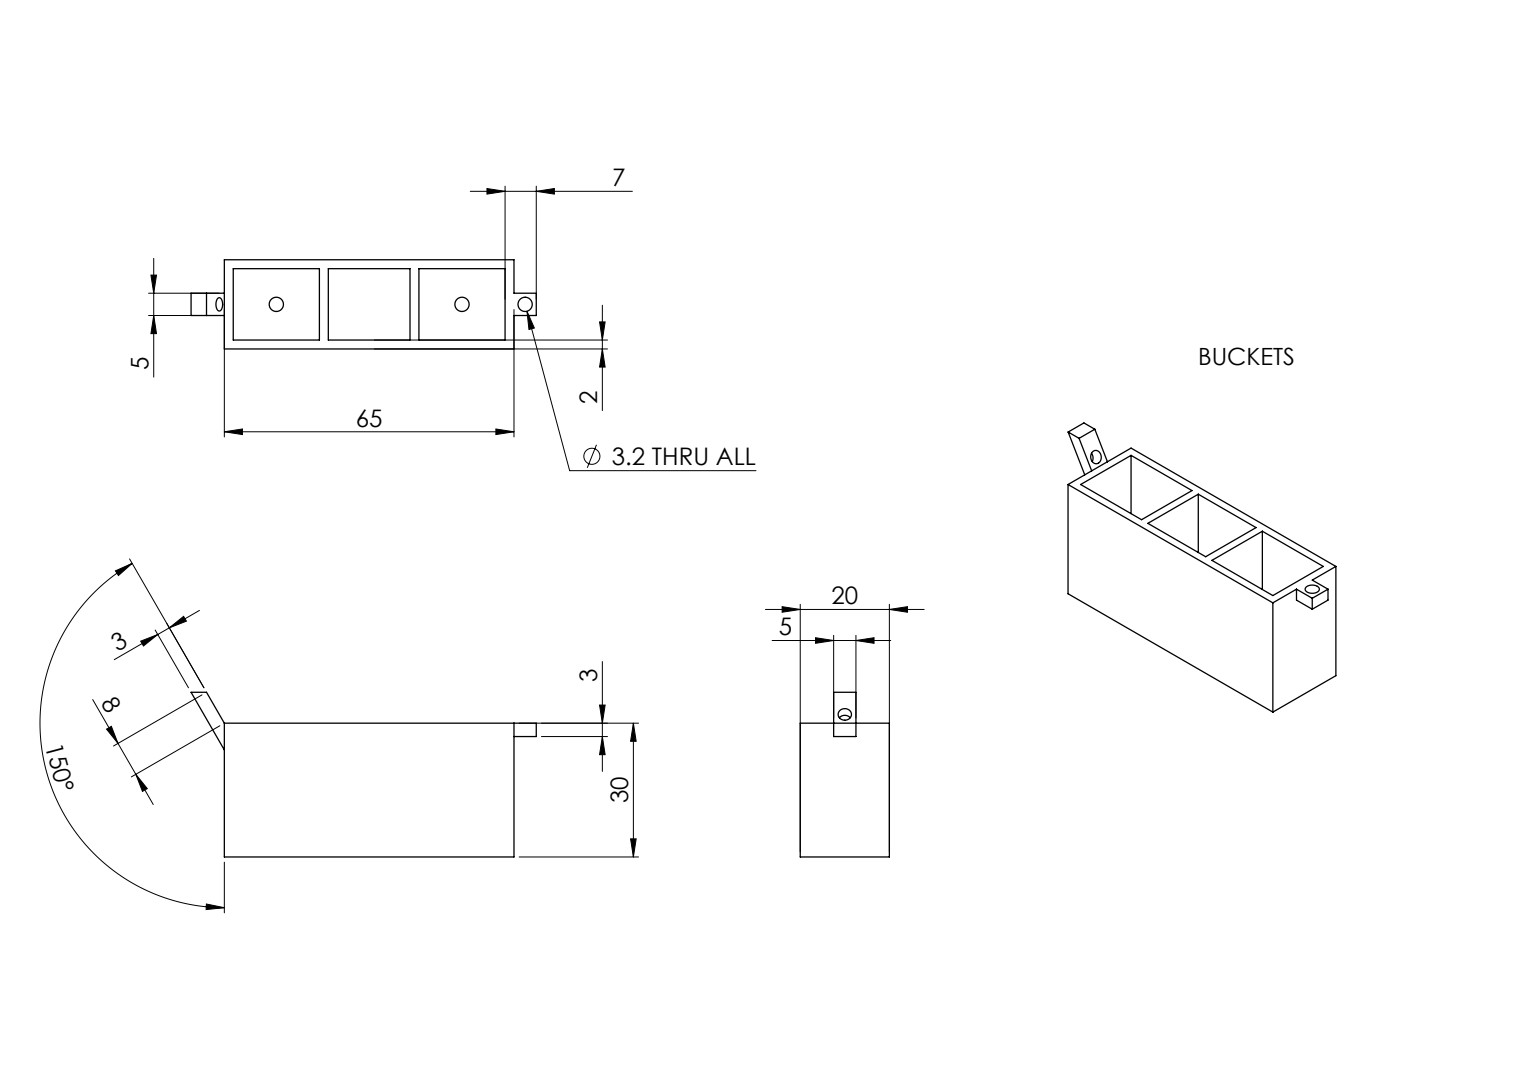
ISO-10303-21;
HEADER;
FILE_DESCRIPTION (('STEP AP214'),
    '1' );
FILE_NAME ('buckets.step',
    '2026-10-26T05:17:54',
    ( '' ),
    ( '' ),
    'SwSTEP 2.0',
    'SolidWorks 2026',
    '' );
FILE_SCHEMA (( 'AUTOMOTIVE_DESIGN' ));
ENDSEC;

DATA;
#10=VECTOR ( 'NONE', #6065, 1000.000000000000000 ) ;
#11=CARTESIAN_POINT ( 'NONE',  ( -6.666666666666660745, 2.000000000000001332, 1.599999999999986766 ) ) ;
#16=EDGE_CURVE ( 'NONE', #1898, #4275, #11568, .T. ) ;
#53=FACE_OUTER_BOUND ( 'NONE', #7053, .T. ) ;
#59=EDGE_CURVE ( 'NONE', #10107, #9996, #12197, .T. ) ;
#63=DIRECTION ( 'NONE',  ( 0.000000000000000000, 0.000000000000000000, 1.000000000000000000 ) ) ;
#76=AXIS2_PLACEMENT_3D ( 'NONE', #9120, #143, #2199 ) ;
#79=CARTESIAN_POINT ( 'NONE',  ( 9.999999999999994671, 27.00000000000000000, -2.500000000000000000 ) ) ;
#89=CARTESIAN_POINT ( 'NONE',  ( -63.73205080756886076, 30.46410161513775350, 0.000000000000000000 ) ) ;
#93=DIRECTION ( 'NONE',  ( -1.000000000000000000, 0.000000000000000000, -5.337610695313252124E-17 ) ) ;
#101=CYLINDRICAL_SURFACE ( 'NONE', #2852, 1.500000000000002665 ) ;
#104=ORIENTED_EDGE ( 'NONE', *, *, #6904, .F. ) ;
#116=ORIENTED_EDGE ( 'NONE', *, *, #12848, .F. ) ;
#143=DIRECTION ( 'NONE',  ( 0.8660254037844394848, 0.4999999999999985012, -0.000000000000000000 ) ) ;
#148=VECTOR ( 'NONE', #2125, 1000.000000000000000 ) ;
#152=( NAMED_UNIT ( * ) SI_UNIT ( $, .STERADIAN. ) SOLID_ANGLE_UNIT ( ) );
#153=DIRECTION ( 'NONE',  ( 1.000000000000000000, 0.000000000000000000, 0.000000000000000000 ) ) ;
#154=CARTESIAN_POINT ( 'NONE',  ( -16.33333333333332504, 2.000000000000000000, -7.999999999999996447 ) ) ;
#177=AXIS2_PLACEMENT_3D ( 'NONE', #10077, #4014, #1048 ) ;
#192=LINE ( 'NONE', #5111, #8966 ) ;
#205=AXIS2_PLACEMENT_3D ( 'NONE', #12610, #4630, #6775 ) ;
#217=FILL_AREA_STYLE ('',( #283 ) ) ;
#220=LINE ( 'NONE', #6117, #2380 ) ;
#231=VECTOR ( 'NONE', #9140, 1000.000000000000000 ) ;
#256=DIRECTION ( 'NONE',  ( 0.000000000000000000, 0.000000000000000000, 1.000000000000000000 ) ) ;
#273=CARTESIAN_POINT ( 'NONE',  ( -60.00000000000000000, 23.99999999999998934, 2.500000000000000000 ) ) ;
#283=FILL_AREA_STYLE_COLOUR ( '', #7592 ) ;
#286=FACE_OUTER_BOUND ( 'NONE', #5183, .T. ) ;
#289=EDGE_LOOP ( 'NONE', ( #1284, #1485, #7281, #1532 ) ) ;
#319=LINE ( 'NONE', #8516, #3101 ) ;
#347=DIRECTION ( 'NONE',  ( -0.000000000000000000, 1.000000000000000000, -0.000000000000000000 ) ) ;
#351=ADVANCED_FACE ( 'NONE', ( #11353 ), #2405, .T. ) ;
#357=DIRECTION ( 'NONE',  ( -1.000000000000000000, -0.000000000000000000, -0.000000000000000000 ) ) ;
#378=ORIENTED_EDGE ( 'NONE', *, *, #6492, .T. ) ;
#381=FACE_BOUND ( 'NONE', #9201, .T. ) ;
#386=DIRECTION ( 'NONE',  ( -0.000000000000000000, 1.000000000000000000, -0.000000000000000000 ) ) ;
#406=LINE ( 'NONE', #4420, #3286 ) ;
#419=EDGE_CURVE ( 'NONE', #6987, #1436, #9061, .T. ) ;
#436=ORIENTED_EDGE ( 'NONE', *, *, #12848, .T. ) ;
#445=ORIENTED_EDGE ( 'NONE', *, *, #1486, .T. ) ;
#446=CARTESIAN_POINT ( 'NONE',  ( 0.000000000000000000, 2.000000000000000000, 0.000000000000000000 ) ) ;
#448=VECTOR ( 'NONE', #5301, 1000.000000000000000 ) ;
#449=ORIENTED_EDGE ( 'NONE', *, *, #16, .T. ) ;
#452=DIRECTION ( 'NONE',  ( -0.000000000000000000, -1.000000000000000000, -0.000000000000000000 ) ) ;
#498=ORIENTED_EDGE ( 'NONE', *, *, #4803, .F. ) ;
#513=ORIENTED_EDGE ( 'NONE', *, *, #12102, .F. ) ;
#524=ORIENTED_EDGE ( 'NONE', *, *, #12861, .T. ) ;
#533=VECTOR ( 'NONE', #6646, 1000.000000000000000 ) ;
#534=DIRECTION ( 'NONE',  ( 0.4999999999999987232, -0.8660254037844393737, 0.000000000000000000 ) ) ;
#544=LINE ( 'NONE', #8546, #10 ) ;
#551=DIRECTION ( 'NONE',  ( -0.000000000000000000, -1.000000000000000000, -0.000000000000000000 ) ) ;
#569=AXIS2_PLACEMENT_3D ( 'NONE', #2591, #4682, #2724 ) ;
#573=SHAPE_DEFINITION_REPRESENTATION ( #2509, #985 ) ;
#585=VERTEX_POINT ( 'NONE', #1932 ) ;
#590=ORIENTED_EDGE ( 'NONE', *, *, #5677, .T. ) ;
#597=DIRECTION ( 'NONE',  ( -0.000000000000000000, -1.000000000000000000, -0.000000000000000000 ) ) ;
#604=CARTESIAN_POINT ( 'NONE',  ( -6.666666666666660745, 2.000000000000001332, -1.599999999999986766 ) ) ;
#605=VECTOR ( 'NONE', #12118, 1000.000000000000000 ) ;
#608=VECTOR ( 'NONE', #6526, 1000.000000000000000 ) ;
#616=VECTOR ( 'NONE', #1823, 1000.000000000000000 ) ;
#635=DIRECTION ( 'NONE',  ( -1.000000000000000000, 0.000000000000000000, 0.000000000000000000 ) ) ;
#637=DIRECTION ( 'NONE',  ( 0.000000000000000000, 0.000000000000000000, -1.000000000000000000 ) ) ;
#649=LINE ( 'NONE', #2821, #9778 ) ;
#654=CARTESIAN_POINT ( 'NONE',  ( -60.00000000000000000, 30.00000000000000000, 2.500000000000000000 ) ) ;
#669=VECTOR ( 'NONE', #1046, 1000.000000000000000 ) ;
#677=VECTOR ( 'NONE', #9665, 1000.000000000000000 ) ;
#688=CARTESIAN_POINT ( 'NONE',  ( 7.500000000000000000, 27.00000000000000000, 0.000000000000000000 ) ) ;
#697=CARTESIAN_POINT ( 'NONE',  ( 0.000000000000000000, 2.000000000000000000, 0.000000000000000000 ) ) ;
#703=VERTEX_POINT ( 'NONE', #4159 ) ;
#712=LINE ( 'NONE', #12759, #4156 ) ;
#720=EDGE_LOOP ( 'NONE', ( #4308, #11552, #5164, #9758 ) ) ;
#727=CARTESIAN_POINT ( 'NONE',  ( -60.00000000000000000, 30.00000000000000000, 9.999999999999996447 ) ) ;
#734=CIRCLE ( 'NONE', #6785, 1.599999999999997202 ) ;
#747=EDGE_CURVE ( 'NONE', #10649, #11707, #5061, .T. ) ;
#751=CARTESIAN_POINT ( 'NONE',  ( 5.000000000000004441, 30.00000000000000000, -2.500000000000000444 ) ) ;
#762=DIRECTION ( 'NONE',  ( -0.000000000000000000, -1.000000000000000000, -0.000000000000000000 ) ) ;
#764=DIRECTION ( 'NONE',  ( -1.000000000000000000, 0.000000000000000000, 0.000000000000000000 ) ) ;
#774=ADVANCED_FACE ( 'NONE', ( #8212, #1329 ), #3249, .F. ) ;
#782=ORIENTED_EDGE ( 'NONE', *, *, #419, .T. ) ;
#788=DIRECTION ( 'NONE',  ( -0.000000000000000000, 1.000000000000000000, -0.000000000000000000 ) ) ;
#792=CIRCLE ( 'NONE', #10416, 1.599999999999992095 ) ;
#793=CARTESIAN_POINT ( 'NONE',  ( -57.99999999999999289, 30.00000000000000000, -8.000000000000003553 ) ) ;
#794=EDGE_CURVE ( 'NONE', #11167, #1351, #9250, .T. ) ;
#826=DIRECTION ( 'NONE',  ( 0.5000000000000005551, -0.8660254037844383745, 0.000000000000000000 ) ) ;
#846=EDGE_LOOP ( 'NONE', ( #6406, #7183, #10691, #3671 ) ) ;
#848=CARTESIAN_POINT ( 'NONE',  ( 0.000000000000000000, 2.000000000000000000, 0.000000000000000000 ) ) ;
#861=EDGE_LOOP ( 'NONE', ( #5404, #2432, #3556, #8105 ) ) ;
#876=CARTESIAN_POINT ( 'NONE',  ( -38.66666666666665719, 30.00000000000000000, -7.999999999999996447 ) ) ;
#884=LINE ( 'NONE', #4888, #12292 ) ;
#895=EDGE_CURVE ( 'NONE', #11453, #7103, #8540, .T. ) ;
#899=PLANE ( 'NONE',  #11027 ) ;
#907=ORIENTED_EDGE ( 'NONE', *, *, #8637, .T. ) ;
#915=FACE_OUTER_BOUND ( 'NONE', #12172, .T. ) ;
#919=VERTEX_POINT ( 'NONE', #604 ) ;
#923=LINE ( 'NONE', #4988, #10114 ) ;
#941=AXIS2_PLACEMENT_3D ( 'NONE', #12279, #5334, #12079 ) ;
#944=ORIENTED_EDGE ( 'NONE', *, *, #9425, .F. ) ;
#946=VERTEX_POINT ( 'NONE', #11338 ) ;
#959=ORIENTED_EDGE ( 'NONE', *, *, #12861, .F. ) ;
#985=SHAPE_REPRESENTATION ( 'buckets', ( #5704 ), #1096 ) ;
#994=EDGE_CURVE ( 'NONE', #5904, #1184, #923, .T. ) ;
#1000=CARTESIAN_POINT ( 'NONE',  ( 4.270088556250601699E-16, 30.00000000000000000, -8.000000000000000000 ) ) ;
#1007=DIRECTION ( 'NONE',  ( -0.000000000000000000, 0.000000000000000000, 1.000000000000000000 ) ) ;
#1028=ORIENTED_EDGE ( 'NONE', *, *, #8827, .F. ) ;
#1032=CARTESIAN_POINT ( 'NONE',  ( 3.000000000000004441, 30.00000000000000000, -10.00000000000000000 ) ) ;
#1037=ORIENTED_EDGE ( 'NONE', *, *, #2209, .F. ) ;
#1046=DIRECTION ( 'NONE',  ( -0.000000000000000000, 1.000000000000000000, -0.000000000000000000 ) ) ;
#1048=DIRECTION ( 'NONE',  ( -1.000000000000000000, 0.000000000000000000, -5.337610695313252124E-17 ) ) ;
#1057=ORIENTED_EDGE ( 'NONE', *, *, #4752, .T. ) ;
#1070=STYLED_ITEM('',(#12995),#11791);
#1078=SURFACE_STYLE_FILL_AREA ( #217 ) ;
#1083=ORIENTED_EDGE ( 'NONE', *, *, #11509, .F. ) ;
#1085=DIRECTION ( 'NONE',  ( -0.000000000000000000, -1.000000000000000000, -0.000000000000000000 ) ) ;
#1088=CARTESIAN_POINT ( 'NONE',  ( -63.99999999999998579, 36.92820323027551410, -2.500000000000000000 ) ) ;
#1094=PLANE ( 'NONE',  #2692 ) ;
#1096=( GEOMETRIC_REPRESENTATION_CONTEXT ( 3 ) GLOBAL_UNCERTAINTY_ASSIGNED_CONTEXT ( ( #6479 ) ) GLOBAL_UNIT_ASSIGNED_CONTEXT ( ( #3190, #9328, #152 ) ) REPRESENTATION_CONTEXT ( 'NONE', 'WORKASPACE' ) );
#1117=DIRECTION ( 'NONE',  ( 0.000000000000000000, 1.000000000000000000, 0.000000000000000000 ) ) ;
#1143=EDGE_LOOP ( 'NONE', ( #5966, #12184, #3162, #12895 ) ) ;
#1153=EDGE_CURVE ( 'NONE', #2281, #8808, #11372, .T. ) ;
#1164=DIRECTION ( 'NONE',  ( 0.000000000000000000, 0.000000000000000000, -1.000000000000000000 ) ) ;
#1184=VERTEX_POINT ( 'NONE', #10716 ) ;
#1221=CARTESIAN_POINT ( 'NONE',  ( -60.38397459621555186, 30.66506350946108128, 0.000000000000000000 ) ) ;
#1228=PLANE ( 'NONE',  #11328 ) ;
#1243=DIRECTION ( 'NONE',  ( -0.000000000000000000, -1.000000000000000000, -0.000000000000000000 ) ) ;
#1247=FACE_BOUND ( 'NONE', #3736, .T. ) ;
#1251=CARTESIAN_POINT ( 'NONE',  ( -48.33333333333332860, 2.000000000000001332, -1.599999999999992095 ) ) ;
#1284=ORIENTED_EDGE ( 'NONE', *, *, #4752, .F. ) ;
#1286=CARTESIAN_POINT ( 'NONE',  ( -61.88397459621555186, 33.26313972081440085, 1.836970198721030427E-16 ) ) ;
#1294=CARTESIAN_POINT ( 'NONE',  ( -60.00000000000000000, 30.00000000000000000, 7.999999999999996447 ) ) ;
#1298=VECTOR ( 'NONE', #9824, 1000.000000000000000 ) ;
#1300=EDGE_LOOP ( 'NONE', ( #9011, #8775, #11719, #6124 ) ) ;
#1305=ORIENTED_EDGE ( 'NONE', *, *, #12229, .T. ) ;
#1309=CARTESIAN_POINT ( 'NONE',  ( 9.999999999999994671, 30.00000000000000000, -2.500000000000000000 ) ) ;
#1312=ORIENTED_EDGE ( 'NONE', *, *, #1891, .T. ) ;
#1319=CARTESIAN_POINT ( 'NONE',  ( -67.46410161513773573, 36.92820323027551410, 2.500000000000000000 ) ) ;
#1329=FACE_OUTER_BOUND ( 'NONE', #9005, .T. ) ;
#1330=DIRECTION ( 'NONE',  ( 1.000000000000000000, 0.000000000000000000, 5.337610695313252124E-17 ) ) ;
#1344=PLANE ( 'NONE',  #941 ) ;
#1350=AXIS2_PLACEMENT_3D ( 'NONE', #2842, #6816, #8722 ) ;
#1351=VERTEX_POINT ( 'NONE', #3602 ) ;
#1365=ORIENTED_EDGE ( 'NONE', *, *, #8234, .T. ) ;
#1376=DIRECTION ( 'NONE',  ( 0.000000000000000000, -1.000000000000000000, -0.000000000000000000 ) ) ;
#1387=DIRECTION ( 'NONE',  ( -0.000000000000000000, 1.000000000000000000, -0.000000000000000000 ) ) ;
#1407=VECTOR ( 'NONE', #3256, 1000.000000000000000 ) ;
#1419=EDGE_LOOP ( 'NONE', ( #8931, #6655, #498, #10152 ) ) ;
#1424=ORIENTED_EDGE ( 'NONE', *, *, #2897, .T. ) ;
#1436=VERTEX_POINT ( 'NONE', #10051 ) ;
#1440=FACE_BOUND ( 'NONE', #6999, .T. ) ;
#1449=LINE ( 'NONE', #9430, #6672 ) ;
#1485=ORIENTED_EDGE ( 'NONE', *, *, #8450, .T. ) ;
#1486=EDGE_CURVE ( 'NONE', #703, #11167, #3922, .T. ) ;
#1491=AXIS2_PLACEMENT_3D ( 'NONE', #12304, #2242, #3156 ) ;
#1492=DIRECTION ( 'NONE',  ( 1.000000000000000000, 0.000000000000000000, 0.000000000000000000 ) ) ;
#1532=ORIENTED_EDGE ( 'NONE', *, *, #4652, .F. ) ;
#1550=EDGE_LOOP ( 'NONE', ( #2996, #1028, #11226, #9089 ) ) ;
#1560=CARTESIAN_POINT ( 'NONE',  ( -36.66666666666665009, 2.000000000000000000, -7.999999999999996447 ) ) ;
#1562=DIRECTION ( 'NONE',  ( 0.000000000000000000, 1.000000000000000000, 0.000000000000000000 ) ) ;
#1575=DIRECTION ( 'NONE',  ( 0.000000000000000000, -1.000000000000000000, 0.000000000000000000 ) ) ;
#1582=AXIS2_PLACEMENT_3D ( 'NONE', #2816, #12754, #6984 ) ;
#1607=CARTESIAN_POINT ( 'NONE',  ( -6.666666666666660745, 2.000000000000000000, 1.599999999999992539 ) ) ;
#1613=VERTEX_POINT ( 'NONE', #3457 ) ;
#1622=ORIENTED_EDGE ( 'NONE', *, *, #5956, .T. ) ;
#1629=DIRECTION ( 'NONE',  ( 0.000000000000000000, -1.000000000000000000, -0.000000000000000000 ) ) ;
#1654=EDGE_CURVE ( 'NONE', #1825, #11750, #10183, .T. ) ;
#1677=EDGE_CURVE ( 'NONE', #2240, #11707, #3586, .T. ) ;
#1691=FACE_OUTER_BOUND ( 'NONE', #4404, .T. ) ;
#1693=CARTESIAN_POINT ( 'NONE',  ( -60.00000000000000000, 30.00000000000000000, 9.999999999999996447 ) ) ;
#1720=AXIS2_PLACEMENT_3D ( 'NONE', #10273, #10210, #7396 ) ;
#1722=DIRECTION ( 'NONE',  ( 0.000000000000000000, -0.000000000000000000, -1.000000000000000000 ) ) ;
#1740=DIRECTION ( 'NONE',  ( 1.000000000000000000, 0.000000000000000000, 0.000000000000000000 ) ) ;
#1768=DIRECTION ( 'NONE',  ( -0.8660254037844394848, -0.4999999999999984457, -0.000000000000000000 ) ) ;
#1772=FACE_OUTER_BOUND ( 'NONE', #2765, .T. ) ;
#1785=VECTOR ( 'NONE', #1740, 1000.000000000000000 ) ;
#1788=CARTESIAN_POINT ( 'NONE',  ( -67.46410161513773573, 36.92820323027551410, -2.500000000000000000 ) ) ;
#1794=CARTESIAN_POINT ( 'NONE',  ( 5.000000000000004441, 30.00000000000000000, 2.500000000000000444 ) ) ;
#1800=DIRECTION ( 'NONE',  ( 1.000000000000000000, 0.000000000000000000, -0.000000000000000000 ) ) ;
#1812=ORIENTED_EDGE ( 'NONE', *, *, #2129, .T. ) ;
#1823=DIRECTION ( 'NONE',  ( 0.000000000000000000, 0.000000000000000000, 1.000000000000000000 ) ) ;
#1825=VERTEX_POINT ( 'NONE', #751 ) ;
#1827=FACE_OUTER_BOUND ( 'NONE', #289, .T. ) ;
#1833=FACE_OUTER_BOUND ( 'NONE', #10045, .T. ) ;
#1834=VECTOR ( 'NONE', #5391, 1000.000000000000000 ) ;
#1847=DIRECTION ( 'NONE',  ( -0.000000000000000000, -1.000000000000000000, -0.000000000000000000 ) ) ;
#1862=VERTEX_POINT ( 'NONE', #11 ) ;
#1880=DIRECTION ( 'NONE',  ( 0.4999999999999995559, -0.8660254037844389297, 0.000000000000000000 ) ) ;
#1881=FACE_OUTER_BOUND ( 'NONE', #9933, .T. ) ;
#1891=EDGE_CURVE ( 'NONE', #7660, #1613, #7888, .T. ) ;
#1898=VERTEX_POINT ( 'NONE', #6834 ) ;
#1932=CARTESIAN_POINT ( 'NONE',  ( -18.33333333333332504, 2.000000000000000000, -8.000000000000001776 ) ) ;
#1934=CARTESIAN_POINT ( 'NONE',  ( 0.000000000000000000, 0.000000000000000000, 2.500000000000000000 ) ) ;
#1945=STYLED_ITEM ( 'NONE', ( #9062 ), #2170 ) ;
#1986=VERTEX_POINT ( 'NONE', #12924 ) ;
#2021=ORIENTED_EDGE ( 'NONE', *, *, #7692, .F. ) ;
#2022=AXIS2_PLACEMENT_3D ( 'NONE', #4342, #7346, #8463 ) ;
#2041=CIRCLE ( 'NONE', #569, 1.599999999999990319 ) ;
#2052=CARTESIAN_POINT ( 'NONE',  ( 5.000000000000004441, 0.000000000000000000, -10.00000000000000000 ) ) ;
#2066=EDGE_CURVE ( 'NONE', #7103, #11106, #12136, .T. ) ;
#2094=EDGE_CURVE ( 'NONE', #919, #1862, #8889, .T. ) ;
#2125=DIRECTION ( 'NONE',  ( 1.000000000000000000, 0.000000000000000000, 5.337610695313252124E-17 ) ) ;
#2129=EDGE_CURVE ( 'NONE', #3989, #3015, #7231, .T. ) ;
#2134=CARTESIAN_POINT ( 'NONE',  ( -60.00000000000000000, 0.000000000000000000, -10.00000000000000355 ) ) ;
#2170=ADVANCED_BREP_SHAPE_REPRESENTATION ( '', ( #11791, #5704 ), #1096 ) ;
#2199=DIRECTION ( 'NONE',  ( -0.4999999999999985012, 0.8660254037844394848, 0.000000000000000000 ) ) ;
#2209=EDGE_CURVE ( 'NONE', #1825, #4500, #9447, .T. ) ;
#2240=VERTEX_POINT ( 'NONE', #10625 ) ;
#2242=DIRECTION ( 'NONE',  ( 5.337610695313252124E-17, 0.000000000000000000, -1.000000000000000000 ) ) ;
#2267=APPLICATION_CONTEXT ( 'automotive_design' ) ;
#2276=( NAMED_UNIT ( * ) PLANE_ANGLE_UNIT ( ) SI_UNIT ( $, .RADIAN. ) );
#2281=VERTEX_POINT ( 'NONE', #11538 ) ;
#2291=DIRECTION ( 'NONE',  ( 5.337610695313252124E-17, 0.000000000000000000, -1.000000000000000000 ) ) ;
#2312=EDGE_LOOP ( 'NONE', ( #11265, #1812, #3367, #4714 ) ) ;
#2343=DIRECTION ( 'NONE',  ( 0.000000000000000000, -1.000000000000000000, 0.000000000000000000 ) ) ;
#2348=AXIS2_PLACEMENT_3D ( 'NONE', #6745, #12651, #12585 ) ;
#2354=ORIENTED_EDGE ( 'NONE', *, *, #2815, .T. ) ;
#2358=ORIENTED_EDGE ( 'NONE', *, *, #794, .T. ) ;
#2380=VECTOR ( 'NONE', #7304, 1000.000000000000000 ) ;
#2382=ADVANCED_FACE ( 'NONE', ( #9770 ), #6819, .F. ) ;
#2391=DIRECTION ( 'NONE',  ( -0.000000000000000000, 1.000000000000000000, -0.000000000000000000 ) ) ;
#2397=DIRECTION ( 'NONE',  ( 0.000000000000000000, -1.000000000000000000, 0.000000000000000000 ) ) ;
#2405=PLANE ( 'NONE',  #4057 ) ;
#2421=CIRCLE ( 'NONE', #11603, 1.500000000000002665 ) ;
#2426=DIRECTION ( 'NONE',  ( 1.000000000000000000, 0.000000000000000000, 5.337610695313252124E-17 ) ) ;
#2432=ORIENTED_EDGE ( 'NONE', *, *, #4273, .F. ) ;
#2433=VECTOR ( 'NONE', #12944, 1000.000000000000000 ) ;
#2436=LINE ( 'NONE', #9227, #6096 ) ;
#2462=ORIENTED_EDGE ( 'NONE', *, *, #7361, .T. ) ;
#2468=CARTESIAN_POINT ( 'NONE',  ( -57.99999999999999289, 30.00000000000000000, 7.999999999999996447 ) ) ;
#2477=CARTESIAN_POINT ( 'NONE',  ( -57.99999999999999289, 30.00000000000000000, 0.000000000000000000 ) ) ;
#2501=VECTOR ( 'NONE', #6851, 1000.000000000000000 ) ;
#2509=PRODUCT_DEFINITION_SHAPE ( 'NONE', 'NONE',  #8584 ) ;
#2518=EDGE_CURVE ( 'NONE', #8071, #9176, #6094, .T. ) ;
#2521=PLANE ( 'NONE',  #10430 ) ;
#2526=ORIENTED_EDGE ( 'NONE', *, *, #6460, .T. ) ;
#2534=CARTESIAN_POINT ( 'NONE',  ( -60.00000000000000000, 30.00000000000000000, 2.500000000000000000 ) ) ;
#2543=VERTEX_POINT ( 'NONE', #2052 ) ;
#2555=ORIENTED_EDGE ( 'NONE', *, *, #5643, .F. ) ;
#2591=CARTESIAN_POINT ( 'NONE',  ( -48.33333333333332860, 2.000000000000001332, -1.734723475976807094E-15 ) ) ;
#2597=ORIENTED_EDGE ( 'NONE', *, *, #1654, .F. ) ;
#2616=CARTESIAN_POINT ( 'NONE',  ( 9.999999999999994671, 27.00000000000000000, 2.500000000000000000 ) ) ;
#2648=ADVANCED_FACE ( 'NONE', ( #8900, #3940 ), #11718, .F. ) ;
#2692=AXIS2_PLACEMENT_3D ( 'NONE', #1032, #9211, #1164 ) ;
#2715=CARTESIAN_POINT ( 'NONE',  ( 3.000000000000004441, 2.000000000000000000, 8.000000000000000000 ) ) ;
#2722=ORIENTED_EDGE ( 'NONE', *, *, #9570, .F. ) ;
#2724=DIRECTION ( 'NONE',  ( 0.000000000000000000, 0.000000000000000000, 1.000000000000000000 ) ) ;
#2735=PLANE ( 'NONE',  #205 ) ;
#2741=CARTESIAN_POINT ( 'NONE',  ( 3.000000000000004441, 30.00000000000000000, -8.000000000000000000 ) ) ;
#2745=DIRECTION ( 'NONE',  ( -0.000000000000000000, -0.000000000000000000, 1.000000000000000000 ) ) ;
#2750=ORIENTED_EDGE ( 'NONE', *, *, #11121, .F. ) ;
#2762=VERTEX_POINT ( 'NONE', #9091 ) ;
#2765=EDGE_LOOP ( 'NONE', ( #11305, #12086, #8046, #11032 ) ) ;
#2769=ADVANCED_FACE ( 'NONE', ( #1881 ), #9000, .F. ) ;
#2775=DIRECTION ( 'NONE',  ( 0.000000000000000000, -1.000000000000000000, 0.000000000000000000 ) ) ;
#2801=CARTESIAN_POINT ( 'NONE',  ( 7.500000000000000000, 27.00000000000000000, 0.000000000000000000 ) ) ;
#2815=EDGE_CURVE ( 'NONE', #1351, #3214, #3788, .T. ) ;
#2816=CARTESIAN_POINT ( 'NONE',  ( 7.500000000000000000, 27.00000000000000000, 0.000000000000000000 ) ) ;
#2821=CARTESIAN_POINT ( 'NONE',  ( -4.270088556250601699E-16, 30.00000000000000000, 8.000000000000000000 ) ) ;
#2824=ORIENTED_EDGE ( 'NONE', *, *, #9974, .T. ) ;
#2830=DIRECTION ( 'NONE',  ( 0.000000000000000000, -1.000000000000000000, -0.000000000000000000 ) ) ;
#2842=CARTESIAN_POINT ( 'NONE',  ( 0.000000000000000000, 0.000000000000000000, 0.000000000000000000 ) ) ;
#2852=AXIS2_PLACEMENT_3D ( 'NONE', #4309, #6196, #9338 ) ;
#2878=VECTOR ( 'NONE', #7793, 1000.000000000000000 ) ;
#2880=CYLINDRICAL_SURFACE ( 'NONE', #1582, 1.599999999999992095 ) ;
#2886=DIRECTION ( 'NONE',  ( 0.000000000000000000, 0.000000000000000000, -1.000000000000000000 ) ) ;
#2892=ORIENTED_EDGE ( 'NONE', *, *, #8557, .F. ) ;
#2897=EDGE_CURVE ( 'NONE', #1898, #585, #10897, .T. ) ;
#2898=CARTESIAN_POINT ( 'NONE',  ( -64.48205080756885366, 31.76313972081441150, 1.836970198721030427E-16 ) ) ;
#2906=DIRECTION ( 'NONE',  ( -1.000000000000000000, 0.000000000000000000, -5.337610695313252124E-17 ) ) ;
#2913=ORIENTED_EDGE ( 'NONE', *, *, #12321, .F. ) ;
#2936=FACE_OUTER_BOUND ( 'NONE', #9647, .T. ) ;
#2948=ORIENTED_EDGE ( 'NONE', *, *, #9418, .F. ) ;
#2960=PLANE ( 'NONE',  #4438 ) ;
#2964=EDGE_CURVE ( 'NONE', #8808, #5624, #220, .T. ) ;
#2965=ORIENTED_EDGE ( 'NONE', *, *, #12332, .F. ) ;
#2981=CARTESIAN_POINT ( 'NONE',  ( -4.270088556250601699E-16, 30.00000000000000000, 8.000000000000000000 ) ) ;
#2988=CARTESIAN_POINT ( 'NONE',  ( 5.000000000000004441, 0.000000000000000000, 10.00000000000000000 ) ) ;
#2994=CARTESIAN_POINT ( 'NONE',  ( -61.13397459621555186, 31.96410161513774284, 0.000000000000000000 ) ) ;
#2996=ORIENTED_EDGE ( 'NONE', *, *, #12229, .F. ) ;
#3013=ORIENTED_EDGE ( 'NONE', *, *, #10275, .F. ) ;
#3015=VERTEX_POINT ( 'NONE', #154 ) ;
#3022=FACE_BOUND ( 'NONE', #6719, .T. ) ;
#3039=VERTEX_POINT ( 'NONE', #7043 ) ;
#3067=ORIENTED_EDGE ( 'NONE', *, *, #9983, .F. ) ;
#3073=ADVANCED_FACE ( 'NONE', ( #286 ), #1344, .T. ) ;
#3075=ORIENTED_EDGE ( 'NONE', *, *, #9857, .T. ) ;
#3079=VERTEX_POINT ( 'NONE', #1788 ) ;
#3086=ORIENTED_EDGE ( 'NONE', *, *, #895, .T. ) ;
#3089=DIRECTION ( 'NONE',  ( 0.000000000000000000, 0.000000000000000000, 1.000000000000000000 ) ) ;
#3093=LINE ( 'NONE', #5103, #1298 ) ;
#3101=VECTOR ( 'NONE', #1575, 1000.000000000000000 ) ;
#3111=VECTOR ( 'NONE', #4363, 1000.000000000000000 ) ;
#3124=CIRCLE ( 'NONE', #8956, 1.499999999999999778 ) ;
#3126=DIRECTION ( 'NONE',  ( 0.4999999999999995559, -0.8660254037844389297, 0.000000000000000000 ) ) ;
#3138=ORIENTED_EDGE ( 'NONE', *, *, #9857, .F. ) ;
#3155=VECTOR ( 'NONE', #4880, 1000.000000000000000 ) ;
#3156=DIRECTION ( 'NONE',  ( -1.000000000000000000, 0.000000000000000000, -5.337610695313252124E-17 ) ) ;
#3162=ORIENTED_EDGE ( 'NONE', *, *, #2094, .T. ) ;
#3163=VECTOR ( 'NONE', #1387, 1000.000000000000000 ) ;
#3166=DIRECTION ( 'NONE',  ( 0.000000000000000000, -1.000000000000000000, 0.000000000000000000 ) ) ;
#3168=VERTEX_POINT ( 'NONE', #793 ) ;
#3190=( LENGTH_UNIT ( ) NAMED_UNIT ( * ) SI_UNIT ( .MILLI., .METRE. ) );
#3205=EDGE_CURVE ( 'NONE', #4183, #4549, #6381, .T. ) ;
#3214=VERTEX_POINT ( 'NONE', #2534 ) ;
#3220=ORIENTED_EDGE ( 'NONE', *, *, #6904, .T. ) ;
#3232=LINE ( 'NONE', #4274, #9812 ) ;
#3234=VECTOR ( 'NONE', #4674, 1000.000000000000000 ) ;
#3237=AXIS2_PLACEMENT_3D ( 'NONE', #8158, #7170, #3126 ) ;
#3249=PLANE ( 'NONE',  #76 ) ;
#3256=DIRECTION ( 'NONE',  ( 0.000000000000000000, 0.000000000000000000, -1.000000000000000000 ) ) ;
#3261=DIRECTION ( 'NONE',  ( 0.000000000000000000, -1.000000000000000000, 0.000000000000000000 ) ) ;
#3281=DIRECTION ( 'NONE',  ( -0.8660254037844397068, -0.4999999999999985567, -0.000000000000000000 ) ) ;
#3282=ORIENTED_EDGE ( 'NONE', *, *, #4843, .F. ) ;
#3286=VECTOR ( 'NONE', #9449, 1000.000000000000000 ) ;
#3311=VECTOR ( 'NONE', #10618, 1000.000000000000000 ) ;
#3312=CARTESIAN_POINT ( 'NONE',  ( 9.999999999999994671, 30.00000000000000000, 2.500000000000000000 ) ) ;
#3313=CARTESIAN_POINT ( 'NONE',  ( -6.666666666666660745, 0.000000000000000000, -1.599999999999998090 ) ) ;
#3321=DIRECTION ( 'NONE',  ( -1.000000000000000000, 0.000000000000000000, -5.337610695313252124E-17 ) ) ;
#3327=ORIENTED_EDGE ( 'NONE', *, *, #12071, .F. ) ;
#3335=ADVANCED_FACE ( 'NONE', ( #1827 ), #2880, .F. ) ;
#3341=DIRECTION ( 'NONE',  ( 0.000000000000000000, -1.000000000000000000, 0.000000000000000000 ) ) ;
#3347=ORIENTED_EDGE ( 'NONE', *, *, #10558, .T. ) ;
#3359=EDGE_LOOP ( 'NONE', ( #2722, #6802, #5417, #5440 ) ) ;
#3361=CARTESIAN_POINT ( 'NONE',  ( -48.33333333333332860, 0.000000000000000000, -1.734723475976807094E-15 ) ) ;
#3367=ORIENTED_EDGE ( 'NONE', *, *, #7399, .T. ) ;
#3372=EDGE_CURVE ( 'NONE', #11106, #5904, #4899, .T. ) ;
#3384=PLANE ( 'NONE',  #6419 ) ;
#3392=ORIENTED_EDGE ( 'NONE', *, *, #3205, .T. ) ;
#3398=ORIENTED_EDGE ( 'NONE', *, *, #5677, .F. ) ;
#3406=DIRECTION ( 'NONE',  ( 0.000000000000000000, 0.000000000000000000, 1.000000000000000000 ) ) ;
#3418=ADVANCED_FACE ( 'NONE', ( #7050 ), #101, .F. ) ;
#3422=DIRECTION ( 'NONE',  ( -1.000000000000000000, 0.000000000000000000, -5.337610695313252124E-17 ) ) ;
#3438=FACE_OUTER_BOUND ( 'NONE', #1550, .T. ) ;
#3457=CARTESIAN_POINT ( 'NONE',  ( -38.66666666666665719, 30.00000000000000000, 7.999999999999996447 ) ) ;
#3458=LINE ( 'NONE', #12348, #10863 ) ;
#3470=ORIENTED_EDGE ( 'NONE', *, *, #5652, .F. ) ;
#3471=ORIENTED_EDGE ( 'NONE', *, *, #16, .F. ) ;
#3473=VERTEX_POINT ( 'NONE', #1088 ) ;
#3496=CARTESIAN_POINT ( 'NONE',  ( 5.000000000000004441, 30.00000000000000000, 10.00000000000000000 ) ) ;
#3500=CARTESIAN_POINT ( 'NONE',  ( -57.99999999999999289, 2.000000000000000000, 7.999999999999996447 ) ) ;
#3504=DIRECTION ( 'NONE',  ( -0.8660254037844393737, -0.4999999999999987232, 0.000000000000000000 ) ) ;
#3521=CIRCLE ( 'NONE', #11239, 1.500000000000002665 ) ;
#3529=LINE ( 'NONE', #4636, #677 ) ;
#3556=ORIENTED_EDGE ( 'NONE', *, *, #5161, .T. ) ;
#3586=LINE ( 'NONE', #8737, #1785 ) ;
#3589=FACE_OUTER_BOUND ( 'NONE', #9409, .T. ) ;
#3602=CARTESIAN_POINT ( 'NONE',  ( -60.00000000000000000, 23.99999999999998934, 2.500000000000000000 ) ) ;
#3610=( NAMED_UNIT ( * ) PLANE_ANGLE_UNIT ( ) SI_UNIT ( $, .RADIAN. ) );
#3620=DIRECTION ( 'NONE',  ( -0.000000000000000000, -0.000000000000000000, -1.000000000000000000 ) ) ;
#3656=EDGE_CURVE ( 'NONE', #7660, #3168, #7634, .T. ) ;
#3663=LINE ( 'NONE', #9607, #608 ) ;
#3667=LINE ( 'NONE', #9859, #2501 ) ;
#3670=CARTESIAN_POINT ( 'NONE',  ( -60.00000000000000000, 23.99999999999998934, -2.500000000000000000 ) ) ;
#3671=ORIENTED_EDGE ( 'NONE', *, *, #7104, .T. ) ;
#3674=EDGE_CURVE ( 'NONE', #5295, #2281, #8425, .T. ) ;
#3678=VECTOR ( 'NONE', #12166, 1000.000000000000000 ) ;
#3685=VECTOR ( 'NONE', #6965, 1000.000000000000000 ) ;
#3723=EDGE_CURVE ( 'NONE', #1862, #919, #9954, .T. ) ;
#3731=LINE ( 'NONE', #3794, #6887 ) ;
#3734=ORIENTED_EDGE ( 'NONE', *, *, #5652, .T. ) ;
#3736=EDGE_LOOP ( 'NONE', ( #11765, #10718, #6111, #12335 ) ) ;
#3743=DIRECTION ( 'NONE',  ( 0.000000000000000000, 0.000000000000000000, 1.000000000000000000 ) ) ;
#3788=LINE ( 'NONE', #5989, #10306 ) ;
#3794=CARTESIAN_POINT ( 'NONE',  ( -60.00000000000000000, 0.000000000000000000, -10.00000000000000355 ) ) ;
#3811=VERTEX_POINT ( 'NONE', #2134 ) ;
#3812=CYLINDRICAL_SURFACE ( 'NONE', #5256, 1.599999999999992539 ) ;
#3813=CARTESIAN_POINT ( 'NONE',  ( 5.000000000000004441, 0.000000000000000000, -10.00000000000000000 ) ) ;
#3824=AXIS2_PLACEMENT_3D ( 'NONE', #1294, #2291, #5284 ) ;
#3843=CARTESIAN_POINT ( 'NONE',  ( 7.500000000000000000, 27.00000000000000000, -1.599999999999992095 ) ) ;
#3857=DIRECTION ( 'NONE',  ( -1.000000000000000000, -0.000000000000000000, -0.000000000000000000 ) ) ;
#3914=AXIS2_PLACEMENT_3D ( 'NONE', #688, #9538, #4698 ) ;
#3917=DIRECTION ( 'NONE',  ( 1.000000000000000000, 0.000000000000000000, 5.337610695313252124E-17 ) ) ;
#3922=LINE ( 'NONE', #7046, #7424 ) ;
#3938=CARTESIAN_POINT ( 'NONE',  ( -36.66666666666665009, 46.12451549659709116, 7.999999999999996447 ) ) ;
#3940=FACE_OUTER_BOUND ( 'NONE', #846, .T. ) ;
#3946=CARTESIAN_POINT ( 'NONE',  ( -6.666666666666660745, 2.000000000000000000, -1.599999999999992539 ) ) ;
#3960=ORIENTED_EDGE ( 'NONE', *, *, #9679, .T. ) ;
#3965=EDGE_CURVE ( 'NONE', #8608, #3811, #406, .T. ) ;
#3971=DIRECTION ( 'NONE',  ( -0.8660254037844394848, -0.4999999999999984457, -0.000000000000000000 ) ) ;
#3989=VERTEX_POINT ( 'NONE', #6501 ) ;
#3990=( NAMED_UNIT ( * ) SI_UNIT ( $, .STERADIAN. ) SOLID_ANGLE_UNIT ( ) );
#4014=DIRECTION ( 'NONE',  ( 5.337610695313252124E-17, 0.000000000000000000, -1.000000000000000000 ) ) ;
#4057=AXIS2_PLACEMENT_3D ( 'NONE', #6383, #5075, #93 ) ;
#4087=ORIENTED_EDGE ( 'NONE', *, *, #8637, .F. ) ;
#4100=LINE ( 'NONE', #10951, #12336 ) ;
#4139=ADVANCED_FACE ( 'NONE', ( #10553 ), #9309, .F. ) ;
#4143=CYLINDRICAL_SURFACE ( 'NONE', #7929, 1.599999999999993872 ) ;
#4145=CIRCLE ( 'NONE', #11251, 1.599999999999986766 ) ;
#4156=VECTOR ( 'NONE', #1768, 1000.000000000000227 ) ;
#4159=CARTESIAN_POINT ( 'NONE',  ( -63.99999999999998579, 36.92820323027551410, 2.500000000000000000 ) ) ;
#4162=VECTOR ( 'NONE', #6493, 1000.000000000000000 ) ;
#4169=( NAMED_UNIT ( * ) SI_UNIT ( $, .STERADIAN. ) SOLID_ANGLE_UNIT ( ) );
#4172=CYLINDRICAL_SURFACE ( 'NONE', #3237, 1.500000000000002665 ) ;
#4181=EDGE_LOOP ( 'NONE', ( #8232, #6734, #4573, #3734 ) ) ;
#4183=VERTEX_POINT ( 'NONE', #3496 ) ;
#4187=ORIENTED_EDGE ( 'NONE', *, *, #2129, .F. ) ;
#4232=EDGE_CURVE ( 'NONE', #2543, #4549, #12710, .T. ) ;
#4233=DIRECTION ( 'NONE',  ( 0.000000000000000000, 0.000000000000000000, -1.000000000000000000 ) ) ;
#4243=LINE ( 'NONE', #6258, #12121 ) ;
#4265=CARTESIAN_POINT ( 'NONE',  ( -60.00000000000000000, 30.00000000000000000, 9.999999999999996447 ) ) ;
#4273=EDGE_CURVE ( 'NONE', #3039, #3811, #12772, .T. ) ;
#4274=CARTESIAN_POINT ( 'NONE',  ( 9.999999999999994671, 27.00000000000000000, -2.500000000000000000 ) ) ;
#4275=VERTEX_POINT ( 'NONE', #5831 ) ;
#4287=CIRCLE ( 'NONE', #10342, 1.599999999999998090 ) ;
#4304=VECTOR ( 'NONE', #551, 1000.000000000000000 ) ;
#4308=ORIENTED_EDGE ( 'NONE', *, *, #4684, .F. ) ;
#4309=CARTESIAN_POINT ( 'NONE',  ( -63.73205080756886076, 30.46410161513775350, 0.000000000000000000 ) ) ;
#4319=CARTESIAN_POINT ( 'NONE',  ( -48.33333333333332860, 0.000000000000000000, -1.734723475976807094E-15 ) ) ;
#4328=PLANE ( 'NONE',  #10492 ) ;
#4342=CARTESIAN_POINT ( 'NONE',  ( 9.999999999999994671, 27.00000000000000000, -2.500000000000000000 ) ) ;
#4357=VERTEX_POINT ( 'NONE', #8964 ) ;
#4363=DIRECTION ( 'NONE',  ( 1.000000000000000000, 0.000000000000000000, 5.337610695313252124E-17 ) ) ;
#4377=CARTESIAN_POINT ( 'NONE',  ( 7.500000000000000000, 30.00000000000000000, 0.000000000000000000 ) ) ;
#4381=AXIS2_PLACEMENT_3D ( 'NONE', #5636, #4660, #3422 ) ;
#4404=EDGE_LOOP ( 'NONE', ( #590, #9688, #5701, #7390, #10772, #12756, #10894, #5883 ) ) ;
#4420=CARTESIAN_POINT ( 'NONE',  ( -60.00000000000000000, 0.000000000000000000, 9.999999999999996447 ) ) ;
#4426=MECHANICAL_DESIGN_GEOMETRIC_PRESENTATION_REPRESENTATION('',(#1070),#7764);
#4438=AXIS2_PLACEMENT_3D ( 'NONE', #4919, #8905, #10925 ) ;
#4446=LINE ( 'NONE', #2616, #7632 ) ;
#4460=CARTESIAN_POINT ( 'NONE',  ( 5.000000000000004441, 27.00000000000000000, -10.00000000000000000 ) ) ;
#4471=LINE ( 'NONE', #10487, #4162 ) ;
#4473=PLANE ( 'NONE',  #9604 ) ;
#4483=EDGE_CURVE ( 'NONE', #4357, #6677, #12483, .T. ) ;
#4487=ORIENTED_EDGE ( 'NONE', *, *, #10221, .T. ) ;
#4489=PRODUCT ( 'buckets', 'buckets', '', ( #8439 ) ) ;
#4495=VERTEX_POINT ( 'NONE', #6712 ) ;
#4500=VERTEX_POINT ( 'NONE', #9466 ) ;
#4538=CARTESIAN_POINT ( 'NONE',  ( 5.000000000000004441, 30.00000000000000000, -10.00000000000000000 ) ) ;
#4549=VERTEX_POINT ( 'NONE', #2988 ) ;
#4550=EDGE_CURVE ( 'NONE', #4275, #1184, #8744, .T. ) ;
#4552=LINE ( 'NONE', #12598, #1834 ) ;
#4554=CIRCLE ( 'NONE', #6626, 1.599999999999992095 ) ;
#4573=ORIENTED_EDGE ( 'NONE', *, *, #4652, .T. ) ;
#4612=DIRECTION ( 'NONE',  ( 0.4999999999999985012, -0.8660254037844394848, -0.000000000000000000 ) ) ;
#4630=DIRECTION ( 'NONE',  ( 1.000000000000000000, 0.000000000000000000, -0.000000000000000000 ) ) ;
#4636=CARTESIAN_POINT ( 'NONE',  ( 3.000000000000004441, 30.00000000000000000, 0.000000000000000000 ) ) ;
#4652=EDGE_CURVE ( 'NONE', #5149, #6677, #12800, .T. ) ;
#4660=DIRECTION ( 'NONE',  ( 5.337610695313252124E-17, 0.000000000000000000, -1.000000000000000000 ) ) ;
#4672=CARTESIAN_POINT ( 'NONE',  ( -16.33333333333332504, 2.000000000000000000, 7.999999999999996447 ) ) ;
#4674=DIRECTION ( 'NONE',  ( 0.000000000000000000, 0.000000000000000000, -1.000000000000000000 ) ) ;
#4682=DIRECTION ( 'NONE',  ( -0.000000000000000000, 1.000000000000000000, -0.000000000000000000 ) ) ;
#4684=EDGE_CURVE ( 'NONE', #1986, #7217, #5136, .T. ) ;
#4686=VECTOR ( 'NONE', #2745, 1000.000000000000000 ) ;
#4698=DIRECTION ( 'NONE',  ( 0.000000000000000000, 0.000000000000000000, -1.000000000000000000 ) ) ;
#4710=DIRECTION ( 'NONE',  ( 1.000000000000000000, 0.000000000000000000, 5.337610695313252124E-17 ) ) ;
#4713=VECTOR ( 'NONE', #2343, 1000.000000000000000 ) ;
#4714=ORIENTED_EDGE ( 'NONE', *, *, #6460, .F. ) ;
#4745=DIRECTION ( 'NONE',  ( 1.000000000000000000, 0.000000000000000000, 5.337610695313252124E-17 ) ) ;
#4752=EDGE_CURVE ( 'NONE', #6664, #5149, #4554, .T. ) ;
#4757=ADVANCED_FACE ( 'NONE', ( #9059 ), #3384, .F. ) ;
#4759=VECTOR ( 'NONE', #4745, 1000.000000000000000 ) ;
#4764=PLANE ( 'NONE',  #12503 ) ;
#4766=ORIENTED_EDGE ( 'NONE', *, *, #7692, .T. ) ;
#4778=AXIS2_PLACEMENT_3D ( 'NONE', #5476, #1492, #7254 ) ;
#4794=EDGE_CURVE ( 'NONE', #8071, #3015, #7363, .T. ) ;
#4797=CARTESIAN_POINT ( 'NONE',  ( 5.000000000000004441, 30.00000000000000000, -10.00000000000000000 ) ) ;
#4803=EDGE_CURVE ( 'NONE', #3214, #703, #10243, .T. ) ;
#4824=DIRECTION ( 'NONE',  ( 0.000000000000000000, 0.000000000000000000, 1.000000000000000000 ) ) ;
#4842=LINE ( 'NONE', #8893, #8940 ) ;
#4843=EDGE_CURVE ( 'NONE', #8608, #4549, #4552, .T. ) ;
#4844=EDGE_CURVE ( 'NONE', #11182, #1862, #11544, .T. ) ;
#4845=EDGE_CURVE ( 'NONE', #1436, #6987, #2041, .T. ) ;
#4850=LINE ( 'NONE', #3938, #6463 ) ;
#4875=VECTOR ( 'NONE', #9306, 1000.000000000000000 ) ;
#4880=DIRECTION ( 'NONE',  ( 0.000000000000000000, 0.000000000000000000, -1.000000000000000000 ) ) ;
#4886=DIRECTION ( 'NONE',  ( 1.000000000000000000, 0.000000000000000000, 0.000000000000000000 ) ) ;
#4888=CARTESIAN_POINT ( 'NONE',  ( -48.33333333333332860, 2.000000000000000000, -1.599999999999995426 ) ) ;
#4899=LINE ( 'NONE', #10786, #2433 ) ;
#4905=DIRECTION ( 'NONE',  ( 5.337610695313252124E-17, 0.000000000000000000, -1.000000000000000000 ) ) ;
#4919=CARTESIAN_POINT ( 'NONE',  ( 3.000000000000004441, 27.00000000000000000, -2.500000000000000000 ) ) ;
#4928=CARTESIAN_POINT ( 'NONE',  ( 0.000000000000000000, 0.000000000000000000, -2.500000000000000000 ) ) ;
#4935=EDGE_LOOP ( 'NONE', ( #513, #11240, #5997, #1037, #104, #7259, #1083, #10148, #5800, #10980 ) ) ;
#4947=CARTESIAN_POINT ( 'NONE',  ( -4.270088556250601699E-16, 2.000000000000000000, 8.000000000000000000 ) ) ;
#4948=ORIENTED_EDGE ( 'NONE', *, *, #7104, .F. ) ;
#4978=LINE ( 'NONE', #6017, #11087 ) ;
#4988=CARTESIAN_POINT ( 'NONE',  ( -18.33333333333332504, 46.12451549659709116, 7.999999999999996447 ) ) ;
#4998=PLANE ( 'NONE',  #11436 ) ;
#4999=ADVANCED_FACE ( 'NONE', ( #9901 ), #4998, .T. ) ;
#5005=DIRECTION ( 'NONE',  ( 1.000000000000000000, 0.000000000000000000, 0.000000000000000000 ) ) ;
#5021=ORIENTED_EDGE ( 'NONE', *, *, #12102, .T. ) ;
#5026=CARTESIAN_POINT ( 'NONE',  ( -62.98205080756885366, 29.16506350946109194, 0.000000000000000000 ) ) ;
#5031=CARTESIAN_POINT ( 'NONE',  ( 7.500000000000000000, 27.00000000000000000, 1.599999999999992095 ) ) ;
#5057=EDGE_CURVE ( 'NONE', #3989, #6204, #11869, .T. ) ;
#5061=LINE ( 'NONE', #79, #11368 ) ;
#5071=SURFACE_SIDE_STYLE ('',( #1078 ) ) ;
#5075=DIRECTION ( 'NONE',  ( 5.337610695313252124E-17, 0.000000000000000000, -1.000000000000000000 ) ) ;
#5103=CARTESIAN_POINT ( 'NONE',  ( -38.66666666666665719, 46.12451549659709116, -7.999999999999996447 ) ) ;
#5111=CARTESIAN_POINT ( 'NONE',  ( 3.000000000000002665, 30.00000000000000000, 8.000000000000000000 ) ) ;
#5136=LINE ( 'NONE', #11220, #7876 ) ;
#5149=VERTEX_POINT ( 'NONE', #10291 ) ;
#5156=ADVANCED_FACE ( 'NONE', ( #7026 ), #6039, .F. ) ;
#5158=VECTOR ( 'NONE', #9915, 1000.000000000000000 ) ;
#5161=EDGE_CURVE ( 'NONE', #3039, #946, #5190, .T. ) ;
#5164=ORIENTED_EDGE ( 'NONE', *, *, #10221, .F. ) ;
#5176=EDGE_LOOP ( 'NONE', ( #2354, #8870, #445, #2358 ) ) ;
#5179=VECTOR ( 'NONE', #153, 1000.000000000000000 ) ;
#5183=EDGE_LOOP ( 'NONE', ( #2913, #10859, #11100, #6574 ) ) ;
#5190=LINE ( 'NONE', #6101, #148 ) ;
#5198=VECTOR ( 'NONE', #1243, 1000.000000000000000 ) ;
#5215=VECTOR ( 'NONE', #3620, 1000.000000000000000 ) ;
#5217=ORIENTED_EDGE ( 'NONE', *, *, #4845, .F. ) ;
#5224=EDGE_LOOP ( 'NONE', ( #2892, #8948 ) ) ;
#5225=VECTOR ( 'NONE', #5607, 1000.000000000000000 ) ;
#5247=ORIENTED_EDGE ( 'NONE', *, *, #4844, .T. ) ;
#5256=AXIS2_PLACEMENT_3D ( 'NONE', #9949, #12042, #3089 ) ;
#5283=ORIENTED_EDGE ( 'NONE', *, *, #747, .F. ) ;
#5284=DIRECTION ( 'NONE',  ( -1.000000000000000000, 0.000000000000000000, -5.337610695313252124E-17 ) ) ;
#5295=VERTEX_POINT ( 'NONE', #3500 ) ;
#5300=CARTESIAN_POINT ( 'NONE',  ( 9.999999999999994671, 27.00000000000000000, 2.500000000000000000 ) ) ;
#5301=DIRECTION ( 'NONE',  ( 1.000000000000000000, 0.000000000000000000, 5.337610695313252124E-17 ) ) ;
#5302=DIRECTION ( 'NONE',  ( 0.000000000000000000, 0.000000000000000000, 1.000000000000000000 ) ) ;
#5304=CARTESIAN_POINT ( 'NONE',  ( -36.66666666666665009, 30.00000000000000000, -7.999999999999996447 ) ) ;
#5314=EDGE_CURVE ( 'NONE', #7217, #3473, #7608, .T. ) ;
#5333=LINE ( 'NONE', #7106, #5179 ) ;
#5334=DIRECTION ( 'NONE',  ( 0.000000000000000000, 0.000000000000000000, 1.000000000000000000 ) ) ;
#5342=EDGE_LOOP ( 'NONE', ( #9076, #3347, #2462, #7249 ) ) ;
#5377=ADVANCED_FACE ( 'NONE', ( #53 ), #9160, .T. ) ;
#5391=DIRECTION ( 'NONE',  ( 1.000000000000000000, 0.000000000000000000, 5.337610695313252124E-17 ) ) ;
#5397=DIRECTION ( 'NONE',  ( 0.000000000000000000, 0.000000000000000000, 1.000000000000000000 ) ) ;
#5404=ORIENTED_EDGE ( 'NONE', *, *, #9909, .F. ) ;
#5414=EDGE_LOOP ( 'NONE', ( #11866, #7784 ) ) ;
#5415=VECTOR ( 'NONE', #12703, 1000.000000000000000 ) ;
#5417=ORIENTED_EDGE ( 'NONE', *, *, #9418, .T. ) ;
#5427=FACE_OUTER_BOUND ( 'NONE', #7555, .T. ) ;
#5433=ORIENTED_EDGE ( 'NONE', *, *, #2209, .T. ) ;
#5440=ORIENTED_EDGE ( 'NONE', *, *, #2518, .F. ) ;
#5476=CARTESIAN_POINT ( 'NONE',  ( 5.000000000000004441, 30.00000000000000000, -10.00000000000000000 ) ) ;
#5485=EDGE_CURVE ( 'NONE', #4500, #7918, #6344, .T. ) ;
#5505=ORIENTED_EDGE ( 'NONE', *, *, #12124, .F. ) ;
#5517=CARTESIAN_POINT ( 'NONE',  ( -60.00000000000000000, 30.00000000000000000, -8.000000000000003553 ) ) ;
#5550=DIRECTION ( 'NONE',  ( -0.000000000000000000, 1.000000000000000000, -0.000000000000000000 ) ) ;
#5564=EDGE_CURVE ( 'NONE', #3168, #2281, #319, .T. ) ;
#5586=VECTOR ( 'NONE', #5658, 1000.000000000000000 ) ;
#5600=ORIENTED_EDGE ( 'NONE', *, *, #9425, .T. ) ;
#5607=DIRECTION ( 'NONE',  ( 0.000000000000000000, 0.000000000000000000, -1.000000000000000000 ) ) ;
#5613=FACE_OUTER_BOUND ( 'NONE', #4181, .T. ) ;
#5617=CARTESIAN_POINT ( 'NONE',  ( -38.66666666666665719, 2.000000000000000000, -7.999999999999996447 ) ) ;
#5624=VERTEX_POINT ( 'NONE', #6799 ) ;
#5636=CARTESIAN_POINT ( 'NONE',  ( -60.00000000000000000, 30.00000000000000000, 7.999999999999996447 ) ) ;
#5643=EDGE_CURVE ( 'NONE', #6259, #10216, #649, .T. ) ;
#5644=LINE ( 'NONE', #4538, #10286 ) ;
#5652=EDGE_CURVE ( 'NONE', #6677, #4357, #4145, .T. ) ;
#5658=DIRECTION ( 'NONE',  ( -0.4999999999999987232, 0.8660254037844393737, 0.000000000000000000 ) ) ;
#5677=EDGE_CURVE ( 'NONE', #1351, #1986, #4842, .T. ) ;
#5690=ORIENTED_EDGE ( 'NONE', *, *, #8588, .F. ) ;
#5701=ORIENTED_EDGE ( 'NONE', *, *, #11509, .T. ) ;
#5704=AXIS2_PLACEMENT_3D ( 'NONE', #8997, #4824, #4886 ) ;
#5737=EDGE_CURVE ( 'NONE', #10107, #12599, #712, .T. ) ;
#5742=AXIS2_PLACEMENT_3D ( 'NONE', #12701, #11843, #3743 ) ;
#5762=VECTOR ( 'NONE', #7682, 1000.000000000000000 ) ;
#5768=ADVANCED_FACE ( 'NONE', ( #1833 ), #899, .F. ) ;
#5771=DIRECTION ( 'NONE',  ( 0.000000000000000000, 0.000000000000000000, 1.000000000000000000 ) ) ;
#5774=PLANE ( 'NONE',  #11681 ) ;
#5800=ORIENTED_EDGE ( 'NONE', *, *, #8822, .F. ) ;
#5815=ADVANCED_FACE ( 'NONE', ( #8108 ), #1094, .F. ) ;
#5817=EDGE_LOOP ( 'NONE', ( #9553, #5690, #5283, #5600 ) ) ;
#5831=CARTESIAN_POINT ( 'NONE',  ( -36.66666666666665009, 2.000000000000000000, 7.999999999999998224 ) ) ;
#5835=VECTOR ( 'NONE', #6748, 1000.000000000000000 ) ;
#5883=ORIENTED_EDGE ( 'NONE', *, *, #2815, .F. ) ;
#5900=VECTOR ( 'NONE', #12556, 1000.000000000000000 ) ;
#5904=VERTEX_POINT ( 'NONE', #10193 ) ;
#5956=EDGE_CURVE ( 'NONE', #5149, #6664, #792, .T. ) ;
#5966=ORIENTED_EDGE ( 'NONE', *, *, #8244, .F. ) ;
#5989=CARTESIAN_POINT ( 'NONE',  ( -60.00000000000000000, 30.00000000000000000, 2.500000000000000000 ) ) ;
#5997=ORIENTED_EDGE ( 'NONE', *, *, #5485, .F. ) ;
#6017=CARTESIAN_POINT ( 'NONE',  ( -60.00000000000000000, 30.00000000000000000, 9.999999999999996447 ) ) ;
#6020=DIRECTION ( 'NONE',  ( 0.000000000000000000, 0.000000000000000000, 1.000000000000000000 ) ) ;
#6039=CYLINDRICAL_SURFACE ( 'NONE', #10196, 1.599999999999993872 ) ;
#6055=ADVANCED_FACE ( 'NONE', ( #7449 ), #11431, .T. ) ;
#6064=ORIENTED_EDGE ( 'NONE', *, *, #12198, .F. ) ;
#6065=DIRECTION ( 'NONE',  ( 0.000000000000000000, -1.000000000000000000, 0.000000000000000000 ) ) ;
#6085=DIRECTION ( 'NONE',  ( -1.000000000000000000, 0.000000000000000000, 0.000000000000000000 ) ) ;
#6091=CARTESIAN_POINT ( 'NONE',  ( -4.270088556250601699E-16, 30.00000000000000000, 8.000000000000000000 ) ) ;
#6094=LINE ( 'NONE', #11263, #4875 ) ;
#6096=VECTOR ( 'NONE', #6282, 1000.000000000000000 ) ;
#6101=CARTESIAN_POINT ( 'NONE',  ( -60.00000000000000000, 30.00000000000000000, -10.00000000000000355 ) ) ;
#6111=ORIENTED_EDGE ( 'NONE', *, *, #8827, .T. ) ;
#6117=CARTESIAN_POINT ( 'NONE',  ( -38.66666666666665719, 2.000000000000000000, -7.999999999999996447 ) ) ;
#6124=ORIENTED_EDGE ( 'NONE', *, *, #4550, .F. ) ;
#6128=FACE_BOUND ( 'NONE', #7571, .T. ) ;
#6135=ORIENTED_EDGE ( 'NONE', *, *, #8244, .T. ) ;
#6184=CARTESIAN_POINT ( 'NONE',  ( 7.500000000000000000, 30.00000000000000000, 0.000000000000000000 ) ) ;
#6185=ORIENTED_EDGE ( 'NONE', *, *, #8234, .F. ) ;
#6190=UNCERTAINTY_MEASURE_WITH_UNIT (LENGTH_MEASURE( 1.000000000000000082E-05 ), #7461, 'distance_accuracy_value', 'NONE');
#6196=DIRECTION ( 'NONE',  ( -0.8660254037844394848, -0.4999999999999984457, -0.000000000000000000 ) ) ;
#6204=VERTEX_POINT ( 'NONE', #2741 ) ;
#6206=ORIENTED_EDGE ( 'NONE', *, *, #11997, .F. ) ;
#6238=ADVANCED_FACE ( 'NONE', ( #5613 ), #9728, .F. ) ;
#6244=DIRECTION ( 'NONE',  ( -0.000000000000000000, -1.000000000000000000, -0.000000000000000000 ) ) ;
#6252=CARTESIAN_POINT ( 'NONE',  ( 4.270088556250601699E-16, 2.000000000000000000, -8.000000000000000000 ) ) ;
#6258=CARTESIAN_POINT ( 'NONE',  ( -36.66666666666665009, 46.12451549659709116, -7.999999999999996447 ) ) ;
#6259=VERTEX_POINT ( 'NONE', #9245 ) ;
#6278=CARTESIAN_POINT ( 'NONE',  ( -38.66666666666665719, 46.12451549659709116, 7.999999999999996447 ) ) ;
#6282=DIRECTION ( 'NONE',  ( 1.000000000000000000, 0.000000000000000000, 0.000000000000000000 ) ) ;
#6327=PLANE ( 'NONE',  #3824 ) ;
#6343=FACE_BOUND ( 'NONE', #8434, .T. ) ;
#6344=LINE ( 'NONE', #1309, #9359 ) ;
#6347=ORIENTED_EDGE ( 'NONE', *, *, #11898, .T. ) ;
#6370=DIRECTION ( 'NONE',  ( 0.000000000000000000, 0.000000000000000000, 1.000000000000000000 ) ) ;
#6381=LINE ( 'NONE', #8355, #4304 ) ;
#6383=CARTESIAN_POINT ( 'NONE',  ( -60.00000000000000000, 30.00000000000000000, -10.00000000000000355 ) ) ;
#6406=ORIENTED_EDGE ( 'NONE', *, *, #2964, .F. ) ;
#6407=PLANE ( 'NONE',  #1491 ) ;
#6414=ORIENTED_EDGE ( 'NONE', *, *, #3723, .T. ) ;
#6416=LINE ( 'NONE', #654, #5215 ) ;
#6419=AXIS2_PLACEMENT_3D ( 'NONE', #9258, #8284, #3321 ) ;
#6438=LINE ( 'NONE', #10435, #231 ) ;
#6460=EDGE_CURVE ( 'NONE', #6204, #2762, #4471, .T. ) ;
#6463=VECTOR ( 'NONE', #9687, 1000.000000000000000 ) ;
#6479=UNCERTAINTY_MEASURE_WITH_UNIT (LENGTH_MEASURE( 1.000000000000000082E-05 ), #3190, 'distance_accuracy_value', 'NONE');
#6480=ORIENTED_EDGE ( 'NONE', *, *, #1654, .T. ) ;
#6492=EDGE_CURVE ( 'NONE', #1613, #5624, #11377, .T. ) ;
#6493=DIRECTION ( 'NONE',  ( 0.000000000000000000, -1.000000000000000000, 0.000000000000000000 ) ) ;
#6494=CARTESIAN_POINT ( 'NONE',  ( -60.00000000000000000, 30.00000000000000000, 2.500000000000000000 ) ) ;
#6498=CARTESIAN_POINT ( 'NONE',  ( 3.000000000000004441, 30.00000000000000000, -2.500000000000000000 ) ) ;
#6501=CARTESIAN_POINT ( 'NONE',  ( -16.33333333333332504, 30.00000000000000000, -7.999999999999996447 ) ) ;
#6504=DIRECTION ( 'NONE',  ( -0.000000000000000000, 1.000000000000000000, -0.000000000000000000 ) ) ;
#6510=CARTESIAN_POINT ( 'NONE',  ( -48.33333333333332860, 2.000000000000001332, -1.734723475976807094E-15 ) ) ;
#6526=DIRECTION ( 'NONE',  ( 1.000000000000000000, 0.000000000000000000, 5.337610695313252124E-17 ) ) ;
#6551=LINE ( 'NONE', #727, #7754 ) ;
#6554=CARTESIAN_POINT ( 'NONE',  ( -6.666666666666660745, 2.000000000000000000, 0.000000000000000000 ) ) ;
#6558=DIRECTION ( 'NONE',  ( -0.8660254037844393737, -0.4999999999999987232, 0.000000000000000000 ) ) ;
#6574=ORIENTED_EDGE ( 'NONE', *, *, #8588, .T. ) ;
#6600=ORIENTED_EDGE ( 'NONE', *, *, #3372, .T. ) ;
#6618=VECTOR ( 'NONE', #1847, 1000.000000000000000 ) ;
#6619=CYLINDRICAL_SURFACE ( 'NONE', #12371, 1.599999999999992539 ) ;
#6621=CARTESIAN_POINT ( 'NONE',  ( 7.500000000000000000, 27.00000000000000000, -1.599999999999986766 ) ) ;
#6626=AXIS2_PLACEMENT_3D ( 'NONE', #6184, #2397, #4233 ) ;
#6630=EDGE_LOOP ( 'NONE', ( #10481, #10907, #9534, #8792 ) ) ;
#6646=DIRECTION ( 'NONE',  ( 0.000000000000000000, 0.000000000000000000, -1.000000000000000000 ) ) ;
#6655=ORIENTED_EDGE ( 'NONE', *, *, #9679, .F. ) ;
#6664=VERTEX_POINT ( 'NONE', #11404 ) ;
#6672=VECTOR ( 'NONE', #452, 1000.000000000000000 ) ;
#6677=VERTEX_POINT ( 'NONE', #6621 ) ;
#6696=ADVANCED_FACE ( 'NONE', ( #10620, #7481 ), #4473, .F. ) ;
#6699=CARTESIAN_POINT ( 'NONE',  ( -36.66666666666665009, 46.12451549659709116, -7.999999999999996447 ) ) ;
#6712=CARTESIAN_POINT ( 'NONE',  ( -38.66666666666665719, 30.00000000000000000, -7.999999999999996447 ) ) ;
#6719=EDGE_LOOP ( 'NONE', ( #1622, #1057 ) ) ;
#6734=ORIENTED_EDGE ( 'NONE', *, *, #5956, .F. ) ;
#6742=ORIENTED_EDGE ( 'NONE', *, *, #747, .T. ) ;
#6745=CARTESIAN_POINT ( 'NONE',  ( -6.666666666666660745, 0.000000000000000000, 0.000000000000000000 ) ) ;
#6748=DIRECTION ( 'NONE',  ( 0.000000000000000000, 0.000000000000000000, 1.000000000000000000 ) ) ;
#6755=CLOSED_SHELL ( 'NONE', ( #9355, #12127, #3335, #3418, #7169, #11601, #9592, #9187, #6959, #2648, #12387, #12288, #5768, #6055, #351, #8162, #12671, #5815, #4757, #8288, #8794, #2769, #5377, #10301, #4999, #6696, #6892, #774, #10605, #2382, #3073, #12269, #4139, #12713, #7484, #6238, #11498, #5156 ) ) ;
#6769=VECTOR ( 'NONE', #8987, 1000.000000000000000 ) ;
#6775=DIRECTION ( 'NONE',  ( -0.000000000000000000, 0.000000000000000000, -1.000000000000000000 ) ) ;
#6785=AXIS2_PLACEMENT_3D ( 'NONE', #4319, #5550, #3406 ) ;
#6786=DIRECTION ( 'NONE',  ( -1.000000000000000000, 0.000000000000000000, -0.000000000000000000 ) ) ;
#6799=CARTESIAN_POINT ( 'NONE',  ( -38.66666666666665719, 2.000000000000000000, 7.999999999999996447 ) ) ;
#6802=ORIENTED_EDGE ( 'NONE', *, *, #5643, .T. ) ;
#6803=AXIS2_PLACEMENT_3D ( 'NONE', #11339, #2391, #6370 ) ;
#6813=FACE_OUTER_BOUND ( 'NONE', #7666, .T. ) ;
#6816=DIRECTION ( 'NONE',  ( 0.000000000000000000, -1.000000000000000000, -0.000000000000000000 ) ) ;
#6819=PLANE ( 'NONE',  #9528 ) ;
#6834=CARTESIAN_POINT ( 'NONE',  ( -36.66666666666665009, 2.000000000000000000, -7.999999999999996447 ) ) ;
#6846=DIRECTION ( 'NONE',  ( -0.000000000000000000, 1.000000000000000000, -0.000000000000000000 ) ) ;
#6851=DIRECTION ( 'NONE',  ( 1.000000000000000000, 0.000000000000000000, 5.337610695313252124E-17 ) ) ;
#6881=CARTESIAN_POINT ( 'NONE',  ( -67.46410161513773573, 36.92820323027551410, 2.500000000000000000 ) ) ;
#6883=PLANE ( 'NONE',  #1350 ) ;
#6887=VECTOR ( 'NONE', #4710, 1000.000000000000000 ) ;
#6892=ADVANCED_FACE ( 'NONE', ( #11918 ), #5774, .F. ) ;
#6904=EDGE_CURVE ( 'NONE', #946, #1825, #10928, .T. ) ;
#6911=DIRECTION ( 'NONE',  ( 0.000000000000000000, 0.000000000000000000, 1.000000000000000000 ) ) ;
#6917=LINE ( 'NONE', #9739, #616 ) ;
#6959=ADVANCED_FACE ( 'NONE', ( #6813 ), #10018, .F. ) ;
#6965=DIRECTION ( 'NONE',  ( 1.000000000000000000, 0.000000000000000000, 5.337610695313252124E-17 ) ) ;
#6967=DIRECTION ( 'NONE',  ( -0.000000000000000000, 1.000000000000000000, -0.000000000000000000 ) ) ;
#6982=VECTOR ( 'NONE', #3261, 1000.000000000000000 ) ;
#6984=DIRECTION ( 'NONE',  ( 0.000000000000000000, 0.000000000000000000, -1.000000000000000000 ) ) ;
#6987=VERTEX_POINT ( 'NONE', #1251 ) ;
#6992=EDGE_LOOP ( 'NONE', ( #12482, #12948, #3471, #3067 ) ) ;
#6999=EDGE_LOOP ( 'NONE', ( #524, #2555, #3138, #7430 ) ) ;
#7007=FACE_OUTER_BOUND ( 'NONE', #8225, .T. ) ;
#7009=FACE_OUTER_BOUND ( 'NONE', #4935, .T. ) ;
#7026=FACE_OUTER_BOUND ( 'NONE', #11313, .T. ) ;
#7043=CARTESIAN_POINT ( 'NONE',  ( -60.00000000000000000, 30.00000000000000000, -10.00000000000000355 ) ) ;
#7046=CARTESIAN_POINT ( 'NONE',  ( -67.46410161513773573, 36.92820323027551410, 2.500000000000000000 ) ) ;
#7050=FACE_OUTER_BOUND ( 'NONE', #5342, .T. ) ;
#7053=EDGE_LOOP ( 'NONE', ( #8164, #6347, #3013, #8169 ) ) ;
#7061=ORIENTED_EDGE ( 'NONE', *, *, #7530, .F. ) ;
#7079=DIRECTION ( 'NONE',  ( -0.000000000000000000, 1.000000000000000000, -0.000000000000000000 ) ) ;
#7081=ORIENTED_EDGE ( 'NONE', *, *, #1677, .F. ) ;
#7103=VERTEX_POINT ( 'NONE', #5304 ) ;
#7104=EDGE_CURVE ( 'NONE', #5295, #5624, #3663, .T. ) ;
#7106=CARTESIAN_POINT ( 'NONE',  ( 3.000000000000004441, 27.00000000000000000, -2.500000000000000000 ) ) ;
#7120=DIRECTION ( 'NONE',  ( -1.000000000000000000, 0.000000000000000000, -0.000000000000000000 ) ) ;
#7140=EDGE_LOOP ( 'NONE', ( #5217, #8831 ) ) ;
#7169=ADVANCED_FACE ( 'NONE', ( #1691 ), #4764, .T. ) ;
#7170=DIRECTION ( 'NONE',  ( -0.8660254037844394848, -0.4999999999999984457, -0.000000000000000000 ) ) ;
#7183=ORIENTED_EDGE ( 'NONE', *, *, #1153, .F. ) ;
#7191=LINE ( 'NONE', #5031, #3678 ) ;
#7217=VERTEX_POINT ( 'NONE', #10590 ) ;
#7231=LINE ( 'NONE', #11215, #10567 ) ;
#7244=EDGE_LOOP ( 'NONE', ( #3282, #9518, #12310, #9235 ) ) ;
#7247=ORIENTED_EDGE ( 'NONE', *, *, #794, .F. ) ;
#7249=ORIENTED_EDGE ( 'NONE', *, *, #5737, .F. ) ;
#7254=DIRECTION ( 'NONE',  ( 0.000000000000000000, 0.000000000000000000, -1.000000000000000000 ) ) ;
#7258=DIRECTION ( 'NONE',  ( 0.4999999999999995559, -0.8660254037844389297, 0.000000000000000000 ) ) ;
#7259=ORIENTED_EDGE ( 'NONE', *, *, #5161, .F. ) ;
#7270=CARTESIAN_POINT ( 'NONE',  ( -18.33333333333332504, 46.12451549659709116, 7.999999999999996447 ) ) ;
#7281=ORIENTED_EDGE ( 'NONE', *, *, #4483, .T. ) ;
#7304=DIRECTION ( 'NONE',  ( -0.000000000000000000, -0.000000000000000000, 1.000000000000000000 ) ) ;
#7321=CARTESIAN_POINT ( 'NONE',  ( -60.00000000000000000, 0.000000000000000000, 9.999999999999996447 ) ) ;
#7323=EDGE_CURVE ( 'NONE', #12128, #6987, #884, .T. ) ;
#7346=DIRECTION ( 'NONE',  ( -1.000000000000000000, 0.000000000000000000, 0.000000000000000000 ) ) ;
#7361=EDGE_CURVE ( 'NONE', #11555, #12599, #3521, .T. ) ;
#7363=LINE ( 'NONE', #8155, #1407 ) ;
#7364=ORIENTED_EDGE ( 'NONE', *, *, #11382, .T. ) ;
#7372=ORIENTED_EDGE ( 'NONE', *, *, #2518, .T. ) ;
#7390=ORIENTED_EDGE ( 'NONE', *, *, #4273, .T. ) ;
#7396=DIRECTION ( 'NONE',  ( -1.000000000000000000, 0.000000000000000000, -0.000000000000000000 ) ) ;
#7399=EDGE_CURVE ( 'NONE', #3015, #2762, #9129, .T. ) ;
#7423=CARTESIAN_POINT ( 'NONE',  ( 9.999999999999994671, 27.00000000000000000, -2.500000000000000000 ) ) ;
#7424=VECTOR ( 'NONE', #3857, 1000.000000000000000 ) ;
#7430=ORIENTED_EDGE ( 'NONE', *, *, #5057, .T. ) ;
#7432=CARTESIAN_POINT ( 'NONE',  ( -60.00000000000000000, 30.00000000000000000, 9.999999999999996447 ) ) ;
#7435=EDGE_CURVE ( 'NONE', #11750, #10649, #5333, .T. ) ;
#7444=ORIENTED_EDGE ( 'NONE', *, *, #2066, .T. ) ;
#7449=FACE_OUTER_BOUND ( 'NONE', #8357, .T. ) ;
#7454=CARTESIAN_POINT ( 'NONE',  ( 4.270088556250601699E-16, 2.000000000000000000, -8.000000000000000000 ) ) ;
#7461=( LENGTH_UNIT ( ) NAMED_UNIT ( * ) SI_UNIT ( .MILLI., .METRE. ) );
#7481=FACE_OUTER_BOUND ( 'NONE', #1419, .T. ) ;
#7484=ADVANCED_FACE ( 'NONE', ( #9330 ), #4172, .F. ) ;
#7528=CARTESIAN_POINT ( 'NONE',  ( 5.000000000000004441, 27.00000000000000000, -2.500000000000000000 ) ) ;
#7530=EDGE_CURVE ( 'NONE', #7660, #5295, #12212, .T. ) ;
#7555=EDGE_LOOP ( 'NONE', ( #12890, #7372, #2021, #9841 ) ) ;
#7564=DIRECTION ( 'NONE',  ( -0.000000000000000000, 1.000000000000000000, -0.000000000000000000 ) ) ;
#7571=EDGE_LOOP ( 'NONE', ( #3470, #12143 ) ) ;
#7592=COLOUR_RGB ( '',0.8941176470588234615, 0.8941176470588234615, 0.8941176470588234615 ) ;
#7607=CARTESIAN_POINT ( 'NONE',  ( 5.000000000000004441, 30.00000000000000000, -10.00000000000000000 ) ) ;
#7608=LINE ( 'NONE', #8596, #3311 ) ;
#7632=VECTOR ( 'NONE', #1562, 1000.000000000000000 ) ;
#7634=LINE ( 'NONE', #2477, #533 ) ;
#7638=VERTEX_POINT ( 'NONE', #7432 ) ;
#7646=ORIENTED_EDGE ( 'NONE', *, *, #7435, .T. ) ;
#7660=VERTEX_POINT ( 'NONE', #2468 ) ;
#7666=EDGE_LOOP ( 'NONE', ( #7824, #8899, #1424, #12224 ) ) ;
#7672=FACE_OUTER_BOUND ( 'NONE', #1143, .T. ) ;
#7678=CARTESIAN_POINT ( 'NONE',  ( -61.13397459621555186, 31.96410161513774284, 0.000000000000000000 ) ) ;
#7682=DIRECTION ( 'NONE',  ( 1.000000000000000000, 0.000000000000000000, 0.000000000000000000 ) ) ;
#7692=EDGE_CURVE ( 'NONE', #2762, #9176, #9715, .T. ) ;
#7754=VECTOR ( 'NONE', #10552, 1000.000000000000000 ) ;
#7764=( GEOMETRIC_REPRESENTATION_CONTEXT ( 3 ) GLOBAL_UNCERTAINTY_ASSIGNED_CONTEXT ( ( #6190 ) ) GLOBAL_UNIT_ASSIGNED_CONTEXT ( ( #7461, #3610, #3990 ) ) REPRESENTATION_CONTEXT ( 'NONE', 'WORKASPACE' ) );
#7784=ORIENTED_EDGE ( 'NONE', *, *, #9147, .T. ) ;
#7793=DIRECTION ( 'NONE',  ( 0.000000000000000000, 0.000000000000000000, 1.000000000000000000 ) ) ;
#7824=ORIENTED_EDGE ( 'NONE', *, *, #2066, .F. ) ;
#7825=VECTOR ( 'NONE', #9562, 1000.000000000000000 ) ;
#7826=DIRECTION ( 'NONE',  ( -0.000000000000000000, -1.000000000000000000, -0.000000000000000000 ) ) ;
#7844=VECTOR ( 'NONE', #1330, 1000.000000000000000 ) ;
#7876=VECTOR ( 'NONE', #347, 1000.000000000000000 ) ;
#7888=LINE ( 'NONE', #2981, #3685 ) ;
#7918=VERTEX_POINT ( 'NONE', #3312 ) ;
#7922=DIRECTION ( 'NONE',  ( -1.000000000000000000, 0.000000000000000000, -0.000000000000000000 ) ) ;
#7929=AXIS2_PLACEMENT_3D ( 'NONE', #10282, #7079, #256 ) ;
#7975=CARTESIAN_POINT ( 'NONE',  ( -48.33333333333332860, 0.000000000000000000, 1.599999999999995426 ) ) ;
#8046=ORIENTED_EDGE ( 'NONE', *, *, #3656, .F. ) ;
#8069=ORIENTED_EDGE ( 'NONE', *, *, #3723, .F. ) ;
#8071=VERTEX_POINT ( 'NONE', #4672 ) ;
#8084=CARTESIAN_POINT ( 'NONE',  ( 4.270088556250601699E-16, 30.00000000000000000, -8.000000000000000000 ) ) ;
#8103=APPLICATION_CONTEXT ( 'automotive_design' ) ;
#8105=ORIENTED_EDGE ( 'NONE', *, *, #12071, .T. ) ;
#8108=FACE_OUTER_BOUND ( 'NONE', #11882, .T. ) ;
#8146=AXIS2_PLACEMENT_3D ( 'NONE', #3361, #9036, #63 ) ;
#8155=CARTESIAN_POINT ( 'NONE',  ( -16.33333333333332504, 2.000000000000000000, 7.999999999999996447 ) ) ;
#8156=ORIENTED_EDGE ( 'NONE', *, *, #9390, .T. ) ;
#8158=CARTESIAN_POINT ( 'NONE',  ( -63.73205080756886076, 30.46410161513775350, 0.000000000000000000 ) ) ;
#8162=ADVANCED_FACE ( 'NONE', ( #12779, #12905, #11794 ), #6883, .T. ) ;
#8164=ORIENTED_EDGE ( 'NONE', *, *, #3372, .F. ) ;
#8169=ORIENTED_EDGE ( 'NONE', *, *, #994, .F. ) ;
#8174=ORIENTED_EDGE ( 'NONE', *, *, #4232, .F. ) ;
#8200=EDGE_LOOP ( 'NONE', ( #907, #8156 ) ) ;
#8212=FACE_BOUND ( 'NONE', #5224, .T. ) ;
#8220=CARTESIAN_POINT ( 'NONE',  ( -57.99999999999999289, 30.00000000000000000, 7.999999999999996447 ) ) ;
#8225=EDGE_LOOP ( 'NONE', ( #6064, #5505, #5247, #6414 ) ) ;
#8231=ORIENTED_EDGE ( 'NONE', *, *, #9402, .F. ) ;
#8232=ORIENTED_EDGE ( 'NONE', *, *, #8450, .F. ) ;
#8234=EDGE_CURVE ( 'NONE', #2240, #11750, #8519, .T. ) ;
#8244=EDGE_CURVE ( 'NONE', #9021, #11182, #4287, .T. ) ;
#8284=DIRECTION ( 'NONE',  ( 5.337610695313252124E-17, 0.000000000000000000, -1.000000000000000000 ) ) ;
#8287=SHAPE_REPRESENTATION_RELATIONSHIP ( 'NONE' , 'NONE' ,  #985, #2170 ) ;
#8288=ADVANCED_FACE ( 'NONE', ( #1772 ), #10797, .F. ) ;
#8304=CARTESIAN_POINT ( 'NONE',  ( 0.000000000000000000, 27.00000000000000000, 0.000000000000000000 ) ) ;
#8319=PLANE ( 'NONE',  #1720 ) ;
#8332=ORIENTED_EDGE ( 'NONE', *, *, #10275, .T. ) ;
#8355=CARTESIAN_POINT ( 'NONE',  ( 5.000000000000004441, 30.00000000000000000, 10.00000000000000000 ) ) ;
#8357=EDGE_LOOP ( 'NONE', ( #6206, #5021, #3392, #8174, #3327, #3220, #6480, #6185 ) ) ;
#8386=LINE ( 'NONE', #4265, #448 ) ;
#8423=ORIENTED_EDGE ( 'NONE', *, *, #7323, .F. ) ;
#8425=LINE ( 'NONE', #9598, #11197 ) ;
#8434=EDGE_LOOP ( 'NONE', ( #8069, #8592 ) ) ;
#8439=PRODUCT_CONTEXT ( 'NONE', #8103, 'mechanical' ) ;
#8447=DIRECTION ( 'NONE',  ( -1.000000000000000000, 0.000000000000000000, -0.000000000000000000 ) ) ;
#8450=EDGE_CURVE ( 'NONE', #6664, #4357, #7191, .T. ) ;
#8463=DIRECTION ( 'NONE',  ( 0.000000000000000000, 0.000000000000000000, 1.000000000000000000 ) ) ;
#8500=LINE ( 'NONE', #10455, #5900 ) ;
#8503=ORIENTED_EDGE ( 'NONE', *, *, #9390, .F. ) ;
#8516=CARTESIAN_POINT ( 'NONE',  ( -57.99999999999999289, 30.00000000000000000, -8.000000000000005329 ) ) ;
#8519=LINE ( 'NONE', #4460, #7825 ) ;
#8540=LINE ( 'NONE', #9641, #3234 ) ;
#8546=CARTESIAN_POINT ( 'NONE',  ( 5.000000000000004441, 30.00000000000000000, 2.500000000000000444 ) ) ;
#8557=EDGE_CURVE ( 'NONE', #12599, #11555, #2421, .T. ) ;
#8584=PRODUCT_DEFINITION ( 'UNKNOWN', '', #8658, #12872 ) ;
#8588=EDGE_CURVE ( 'NONE', #11707, #7918, #4446, .T. ) ;
#8589=PLANE ( 'NONE',  #4381 ) ;
#8592=ORIENTED_EDGE ( 'NONE', *, *, #2094, .F. ) ;
#8595=DIRECTION ( 'NONE',  ( 0.000000000000000000, 0.000000000000000000, 1.000000000000000000 ) ) ;
#8596=CARTESIAN_POINT ( 'NONE',  ( -60.00000000000000000, 30.00000000000000000, -2.500000000000000000 ) ) ;
#8608=VERTEX_POINT ( 'NONE', #7321 ) ;
#8637=EDGE_CURVE ( 'NONE', #11833, #12128, #734, .T. ) ;
#8643=DIRECTION ( 'NONE',  ( -0.000000000000000000, -1.000000000000000000, -0.000000000000000000 ) ) ;
#8658=PRODUCT_DEFINITION_FORMATION_WITH_SPECIFIED_SOURCE ( 'ANY', '', #4489, .NOT_KNOWN. ) ;
#8692=CARTESIAN_POINT ( 'NONE',  ( -60.00000000000000000, 30.00000000000000000, 9.999999999999996447 ) ) ;
#8704=DIRECTION ( 'NONE',  ( 1.000000000000000000, 0.000000000000000000, 5.337610695313252124E-17 ) ) ;
#8722=DIRECTION ( 'NONE',  ( -1.000000000000000000, 0.000000000000000000, -0.000000000000000000 ) ) ;
#8726=DIRECTION ( 'NONE',  ( 1.000000000000000000, 0.000000000000000000, 0.000000000000000000 ) ) ;
#8737=CARTESIAN_POINT ( 'NONE',  ( 3.000000000000004441, 27.00000000000000000, 2.500000000000000000 ) ) ;
#8741=LINE ( 'NONE', #876, #3155 ) ;
#8744=LINE ( 'NONE', #4947, #5158 ) ;
#8775=ORIENTED_EDGE ( 'NONE', *, *, #9402, .T. ) ;
#8785=AXIS2_PLACEMENT_3D ( 'NONE', #1934, #1007, #5005 ) ;
#8792=ORIENTED_EDGE ( 'NONE', *, *, #8557, .T. ) ;
#8794=ADVANCED_FACE ( 'NONE', ( #2936 ), #11828, .F. ) ;
#8808=VERTEX_POINT ( 'NONE', #5617 ) ;
#8820=VECTOR ( 'NONE', #597, 1000.000000000000000 ) ;
#8822=EDGE_CURVE ( 'NONE', #7638, #3214, #8881, .T. ) ;
#8827=EDGE_CURVE ( 'NONE', #3168, #4495, #3667, .T. ) ;
#8831=ORIENTED_EDGE ( 'NONE', *, *, #419, .F. ) ;
#8870=ORIENTED_EDGE ( 'NONE', *, *, #4803, .T. ) ;
#8881=LINE ( 'NONE', #1693, #12731 ) ;
#8889=CIRCLE ( 'NONE', #6803, 1.599999999999986766 ) ;
#8893=CARTESIAN_POINT ( 'NONE',  ( -60.00000000000000000, 23.99999999999998934, 2.500000000000000000 ) ) ;
#8896=EDGE_LOOP ( 'NONE', ( #7081, #1365, #7646, #6742 ) ) ;
#8899=ORIENTED_EDGE ( 'NONE', *, *, #9983, .T. ) ;
#8900=FACE_BOUND ( 'NONE', #7140, .T. ) ;
#8903=DIRECTION ( 'NONE',  ( 0.000000000000000000, 0.000000000000000000, -1.000000000000000000 ) ) ;
#8905=DIRECTION ( 'NONE',  ( 0.000000000000000000, 0.000000000000000000, 1.000000000000000000 ) ) ;
#8915=DIRECTION ( 'NONE',  ( -0.000000000000000000, 0.000000000000000000, 1.000000000000000000 ) ) ;
#8931=ORIENTED_EDGE ( 'NONE', *, *, #5314, .T. ) ;
#8937=CARTESIAN_POINT ( 'NONE',  ( 4.270088556250601699E-16, 2.000000000000000000, -8.000000000000000000 ) ) ;
#8940=VECTOR ( 'NONE', #9748, 1000.000000000000000 ) ;
#8943=LINE ( 'NONE', #3670, #10448 ) ;
#8948=ORIENTED_EDGE ( 'NONE', *, *, #7361, .F. ) ;
#8956=AXIS2_PLACEMENT_3D ( 'NONE', #7678, #3504, #11666 ) ;
#8964=CARTESIAN_POINT ( 'NONE',  ( 7.500000000000000000, 27.00000000000000000, 1.599999999999986766 ) ) ;
#8966=VECTOR ( 'NONE', #3166, 1000.000000000000000 ) ;
#8987=DIRECTION ( 'NONE',  ( -0.000000000000000000, 0.000000000000000000, 1.000000000000000000 ) ) ;
#8997=CARTESIAN_POINT ( 'NONE',  ( 0.000000000000000000, 0.000000000000000000, 0.000000000000000000 ) ) ;
#9000=PLANE ( 'NONE',  #9261 ) ;
#9005=EDGE_LOOP ( 'NONE', ( #2824, #3398, #7247, #436 ) ) ;
#9011=ORIENTED_EDGE ( 'NONE', *, *, #9639, .F. ) ;
#9021=VERTEX_POINT ( 'NONE', #3313 ) ;
#9036=DIRECTION ( 'NONE',  ( -0.000000000000000000, 1.000000000000000000, -0.000000000000000000 ) ) ;
#9059=FACE_OUTER_BOUND ( 'NONE', #2312, .T. ) ;
#9061=CIRCLE ( 'NONE', #10736, 1.599999999999990319 ) ;
#9062=PRESENTATION_STYLE_ASSIGNMENT (( #11153 ) ) ;
#9076=ORIENTED_EDGE ( 'NONE', *, *, #9147, .F. ) ;
#9084=CARTESIAN_POINT ( 'NONE',  ( -63.73205080756886076, 30.46410161513775350, 0.000000000000000000 ) ) ;
#9089=ORIENTED_EDGE ( 'NONE', *, *, #1153, .T. ) ;
#9091=CARTESIAN_POINT ( 'NONE',  ( 3.000000000000004441, 2.000000000000000000, -8.000000000000000000 ) ) ;
#9114=CARTESIAN_POINT ( 'NONE',  ( -48.33333333333332860, 2.000000000000000000, -1.734723475976807094E-15 ) ) ;
#9120=CARTESIAN_POINT ( 'NONE',  ( -60.00000000000000000, 23.99999999999998934, 2.500000000000000000 ) ) ;
#9121=AXIS2_PLACEMENT_3D ( 'NONE', #12927, #6967, #11818 ) ;
#9129=LINE ( 'NONE', #6252, #3111 ) ;
#9140=DIRECTION ( 'NONE',  ( -0.000000000000000000, -1.000000000000000000, -0.000000000000000000 ) ) ;
#9147=EDGE_CURVE ( 'NONE', #9996, #10107, #3124, .T. ) ;
#9160=PLANE ( 'NONE',  #12909 ) ;
#9168=FACE_OUTER_BOUND ( 'NONE', #10137, .T. ) ;
#9176=VERTEX_POINT ( 'NONE', #2715 ) ;
#9187=ADVANCED_FACE ( 'NONE', ( #3438 ), #2521, .F. ) ;
#9201=EDGE_LOOP ( 'NONE', ( #8231, #3086, #7444, #6600 ) ) ;
#9211=DIRECTION ( 'NONE',  ( 1.000000000000000000, 0.000000000000000000, 0.000000000000000000 ) ) ;
#9227=CARTESIAN_POINT ( 'NONE',  ( 3.000000000000004441, 30.00000000000000000, 2.500000000000000000 ) ) ;
#9231=EDGE_LOOP ( 'NONE', ( #11897, #6135 ) ) ;
#9235=ORIENTED_EDGE ( 'NONE', *, *, #4232, .T. ) ;
#9245=CARTESIAN_POINT ( 'NONE',  ( -16.33333333333332504, 30.00000000000000000, 7.999999999999996447 ) ) ;
#9250=LINE ( 'NONE', #273, #11582 ) ;
#9258=CARTESIAN_POINT ( 'NONE',  ( -60.00000000000000000, 30.00000000000000000, -8.000000000000003553 ) ) ;
#9260=( LENGTH_UNIT ( ) NAMED_UNIT ( * ) SI_UNIT ( .MILLI., .METRE. ) );
#9261=AXIS2_PLACEMENT_3D ( 'NONE', #12745, #764, #6911 ) ;
#9306=DIRECTION ( 'NONE',  ( 1.000000000000000000, 0.000000000000000000, 5.337610695313252124E-17 ) ) ;
#9309=PLANE ( 'NONE',  #2022 ) ;
#9328=( NAMED_UNIT ( * ) PLANE_ANGLE_UNIT ( ) SI_UNIT ( $, .RADIAN. ) );
#9330=FACE_OUTER_BOUND ( 'NONE', #6630, .T. ) ;
#9338=DIRECTION ( 'NONE',  ( 0.4999999999999995559, -0.8660254037844389297, 0.000000000000000000 ) ) ;
#9340=VECTOR ( 'NONE', #7826, 1000.000000000000000 ) ;
#9355=ADVANCED_FACE ( 'NONE', ( #9168 ), #4143, .F. ) ;
#9359=VECTOR ( 'NONE', #5302, 1000.000000000000000 ) ;
#9370=CARTESIAN_POINT ( 'NONE',  ( -18.33333333333332504, 30.00000000000000000, -7.999999999999996447 ) ) ;
#9390=EDGE_CURVE ( 'NONE', #12128, #11833, #9391, .T. ) ;
#9391=CIRCLE ( 'NONE', #8146, 1.599999999999997202 ) ;
#9402=EDGE_CURVE ( 'NONE', #11453, #5904, #10219, .T. ) ;
#9408=AXIS2_PLACEMENT_3D ( 'NONE', #697, #1629, #6786 ) ;
#9409=EDGE_LOOP ( 'NONE', ( #12644, #12345, #1305, #12010 ) ) ;
#9418=EDGE_CURVE ( 'NONE', #10216, #9176, #192, .T. ) ;
#9425=EDGE_CURVE ( 'NONE', #10649, #4500, #3232, .T. ) ;
#9430=CARTESIAN_POINT ( 'NONE',  ( -16.33333333333332504, 46.12451549659709116, 7.999999999999996447 ) ) ;
#9447=LINE ( 'NONE', #6498, #5762 ) ;
#9449=DIRECTION ( 'NONE',  ( 0.000000000000000000, 0.000000000000000000, -1.000000000000000000 ) ) ;
#9466=CARTESIAN_POINT ( 'NONE',  ( 9.999999999999994671, 30.00000000000000000, -2.500000000000000000 ) ) ;
#9490=UNCERTAINTY_MEASURE_WITH_UNIT (LENGTH_MEASURE( 1.000000000000000082E-05 ), #9260, 'distance_accuracy_value', 'NONE');
#9518=ORIENTED_EDGE ( 'NONE', *, *, #3965, .T. ) ;
#9528=AXIS2_PLACEMENT_3D ( 'NONE', #4928, #8915, #8726 ) ;
#9534=ORIENTED_EDGE ( 'NONE', *, *, #5737, .T. ) ;
#9538=DIRECTION ( 'NONE',  ( -0.000000000000000000, -1.000000000000000000, -0.000000000000000000 ) ) ;
#9553=ORIENTED_EDGE ( 'NONE', *, *, #5485, .T. ) ;
#9554=EDGE_CURVE ( 'NONE', #3214, #7217, #6416, .T. ) ;
#9562=DIRECTION ( 'NONE',  ( 0.000000000000000000, 0.000000000000000000, -1.000000000000000000 ) ) ;
#9570=EDGE_CURVE ( 'NONE', #6259, #8071, #1449, .T. ) ;
#9592=ADVANCED_FACE ( 'NONE', ( #10670 ), #8589, .T. ) ;
#9598=CARTESIAN_POINT ( 'NONE',  ( -57.99999999999999289, 2.000000000000000000, 0.000000000000000000 ) ) ;
#9604=AXIS2_PLACEMENT_3D ( 'NONE', #6494, #6558, #534 ) ;
#9607=CARTESIAN_POINT ( 'NONE',  ( -4.270088556250601699E-16, 2.000000000000000000, 8.000000000000000000 ) ) ;
#9622=CARTESIAN_POINT ( 'NONE',  ( -60.00000000000000000, 30.00000000000000000, 9.999999999999996447 ) ) ;
#9639=EDGE_CURVE ( 'NONE', #11453, #4275, #4850, .T. ) ;
#9641=CARTESIAN_POINT ( 'NONE',  ( -36.66666666666665009, 30.00000000000000000, -7.999999999999996447 ) ) ;
#9647=EDGE_LOOP ( 'NONE', ( #12215, #449, #12394, #8332 ) ) ;
#9665=DIRECTION ( 'NONE',  ( -0.000000000000000000, 0.000000000000000000, 1.000000000000000000 ) ) ;
#9679=EDGE_CURVE ( 'NONE', #703, #3473, #10858, .T. ) ;
#9687=DIRECTION ( 'NONE',  ( -0.000000000000000000, -1.000000000000000000, -0.000000000000000000 ) ) ;
#9688=ORIENTED_EDGE ( 'NONE', *, *, #4684, .T. ) ;
#9715=LINE ( 'NONE', #9780, #6769 ) ;
#9728=CYLINDRICAL_SURFACE ( 'NONE', #9999, 1.599999999999992095 ) ;
#9739=CARTESIAN_POINT ( 'NONE',  ( -16.33333333333332504, 30.00000000000000000, 7.999999999999996447 ) ) ;
#9748=DIRECTION ( 'NONE',  ( -0.000000000000000000, -0.000000000000000000, -1.000000000000000000 ) ) ;
#9758=ORIENTED_EDGE ( 'NONE', *, *, #5314, .F. ) ;
#9770=FACE_OUTER_BOUND ( 'NONE', #720, .T. ) ;
#9778=VECTOR ( 'NONE', #8704, 1000.000000000000000 ) ;
#9780=CARTESIAN_POINT ( 'NONE',  ( 3.000000000000004441, 2.000000000000000000, 0.000000000000000000 ) ) ;
#9812=VECTOR ( 'NONE', #1117, 1000.000000000000000 ) ;
#9824=DIRECTION ( 'NONE',  ( -0.000000000000000000, -1.000000000000000000, -0.000000000000000000 ) ) ;
#9841=ORIENTED_EDGE ( 'NONE', *, *, #7399, .F. ) ;
#9848=CARTESIAN_POINT ( 'NONE',  ( -18.33333333333332504, 2.000000000000000000, 7.999999999999996447 ) ) ;
#9857=EDGE_CURVE ( 'NONE', #3989, #6259, #6917, .T. ) ;
#9859=CARTESIAN_POINT ( 'NONE',  ( 4.270088556250601699E-16, 30.00000000000000000, -8.000000000000000000 ) ) ;
#9864=CIRCLE ( 'NONE', #2348, 1.599999999999998090 ) ;
#9883=LINE ( 'NONE', #3946, #669 ) ;
#9899=ORIENTED_EDGE ( 'NONE', *, *, #4794, .T. ) ;
#9901=FACE_OUTER_BOUND ( 'NONE', #6992, .T. ) ;
#9909=EDGE_CURVE ( 'NONE', #3811, #2543, #3731, .T. ) ;
#9915=DIRECTION ( 'NONE',  ( 1.000000000000000000, 0.000000000000000000, 5.337610695313252124E-17 ) ) ;
#9920=DIRECTION ( 'NONE',  ( -0.8660254037844393737, -0.4999999999999987232, 0.000000000000000000 ) ) ;
#9933=EDGE_LOOP ( 'NONE', ( #4187, #3075, #10584, #9899 ) ) ;
#9949=CARTESIAN_POINT ( 'NONE',  ( -6.666666666666660745, 2.000000000000000000, 0.000000000000000000 ) ) ;
#9954=CIRCLE ( 'NONE', #9121, 1.599999999999986766 ) ;
#9974=EDGE_CURVE ( 'NONE', #3079, #1986, #8943, .T. ) ;
#9975=PLANE ( 'NONE',  #8785 ) ;
#9983=EDGE_CURVE ( 'NONE', #7103, #1898, #4243, .T. ) ;
#9985=DIRECTION ( 'NONE',  ( -0.000000000000000000, 1.000000000000000000, -0.000000000000000000 ) ) ;
#9996=VERTEX_POINT ( 'NONE', #1286 ) ;
#9999=AXIS2_PLACEMENT_3D ( 'NONE', #2801, #762, #12743 ) ;
#10018=PLANE ( 'NONE',  #177 ) ;
#10032=DIRECTION ( 'NONE',  ( 0.000000000000000000, 0.000000000000000000, 1.000000000000000000 ) ) ;
#10045=EDGE_LOOP ( 'NONE', ( #12694, #12164, #2965, #7364 ) ) ;
#10047=DIRECTION ( 'NONE',  ( -0.8660254037844397068, -0.4999999999999985567, -0.000000000000000000 ) ) ;
#10051=CARTESIAN_POINT ( 'NONE',  ( -48.33333333333332860, 2.000000000000001332, 1.599999999999988542 ) ) ;
#10077=CARTESIAN_POINT ( 'NONE',  ( -60.00000000000000000, 30.00000000000000000, -8.000000000000003553 ) ) ;
#10107=VERTEX_POINT ( 'NONE', #1221 ) ;
#10114=VECTOR ( 'NONE', #11667, 1000.000000000000000 ) ;
#10137=EDGE_LOOP ( 'NONE', ( #8503, #11542, #782, #2750 ) ) ;
#10148=ORIENTED_EDGE ( 'NONE', *, *, #9554, .F. ) ;
#10152=ORIENTED_EDGE ( 'NONE', *, *, #9554, .T. ) ;
#10183=LINE ( 'NONE', #12150, #4713 ) ;
#10193=CARTESIAN_POINT ( 'NONE',  ( -18.33333333333332504, 30.00000000000000000, 7.999999999999996447 ) ) ;
#10196=AXIS2_PLACEMENT_3D ( 'NONE', #9114, #11073, #10032 ) ;
#10210=DIRECTION ( 'NONE',  ( 0.000000000000000000, -1.000000000000000000, -0.000000000000000000 ) ) ;
#10216=VERTEX_POINT ( 'NONE', #12478 ) ;
#10219=LINE ( 'NONE', #6091, #605 ) ;
#10221=EDGE_CURVE ( 'NONE', #3473, #3079, #3458, .T. ) ;
#10243=LINE ( 'NONE', #11614, #5586 ) ;
#10273=CARTESIAN_POINT ( 'NONE',  ( 0.000000000000000000, 30.00000000000000000, 0.000000000000000000 ) ) ;
#10275=EDGE_CURVE ( 'NONE', #1184, #585, #11817, .T. ) ;
#10282=CARTESIAN_POINT ( 'NONE',  ( -48.33333333333332860, 2.000000000000000000, -1.734723475976807094E-15 ) ) ;
#10286=VECTOR ( 'NONE', #8595, 1000.000000000000000 ) ;
#10291=CARTESIAN_POINT ( 'NONE',  ( 7.500000000000000000, 30.00000000000000000, -1.599999999999992095 ) ) ;
#10301=ADVANCED_FACE ( 'NONE', ( #3589 ), #2735, .F. ) ;
#10306=VECTOR ( 'NONE', #9985, 1000.000000000000000 ) ;
#10342=AXIS2_PLACEMENT_3D ( 'NONE', #11586, #386, #12508 ) ;
#10397=EDGE_CURVE ( 'NONE', #1613, #4495, #8741, .T. ) ;
#10416=AXIS2_PLACEMENT_3D ( 'NONE', #4377, #3341, #11238 ) ;
#10419=CARTESIAN_POINT ( 'NONE',  ( -6.666666666666660745, 0.000000000000000000, 1.599999999999998090 ) ) ;
#10430=AXIS2_PLACEMENT_3D ( 'NONE', #5517, #12591, #2906 ) ;
#10435=CARTESIAN_POINT ( 'NONE',  ( -18.33333333333332504, 46.12451549659709116, -7.999999999999996447 ) ) ;
#10437=ORIENTED_EDGE ( 'NONE', *, *, #4845, .T. ) ;
#10448=VECTOR ( 'NONE', #11639, 1000.000000000000114 ) ;
#10455=CARTESIAN_POINT ( 'NONE',  ( -67.46410161513773573, 36.92820323027551410, 2.500000000000000000 ) ) ;
#10481=ORIENTED_EDGE ( 'NONE', *, *, #10558, .F. ) ;
#10487=CARTESIAN_POINT ( 'NONE',  ( 3.000000000000002665, 30.00000000000000000, -8.000000000000000000 ) ) ;
#10492=AXIS2_PLACEMENT_3D ( 'NONE', #446, #1376, #8447 ) ;
#10552=DIRECTION ( 'NONE',  ( -0.000000000000000000, -1.000000000000000000, -0.000000000000000000 ) ) ;
#10553=FACE_OUTER_BOUND ( 'NONE', #5817, .T. ) ;
#10558=EDGE_CURVE ( 'NONE', #9996, #11555, #4100, .T. ) ;
#10567=VECTOR ( 'NONE', #6244, 1000.000000000000000 ) ;
#10584=ORIENTED_EDGE ( 'NONE', *, *, #9570, .T. ) ;
#10590=CARTESIAN_POINT ( 'NONE',  ( -60.00000000000000000, 30.00000000000000000, -2.500000000000000000 ) ) ;
#10605=ADVANCED_FACE ( 'NONE', ( #10890 ), #9975, .T. ) ;
#10606=VECTOR ( 'NONE', #6504, 1000.000000000000000 ) ;
#10618=DIRECTION ( 'NONE',  ( -0.4999999999999987232, 0.8660254037844393737, 0.000000000000000000 ) ) ;
#10620=FACE_BOUND ( 'NONE', #5414, .T. ) ;
#10625=CARTESIAN_POINT ( 'NONE',  ( 5.000000000000004441, 27.00000000000000000, 2.500000000000000444 ) ) ;
#10649=VERTEX_POINT ( 'NONE', #7423 ) ;
#10670=FACE_OUTER_BOUND ( 'NONE', #1300, .T. ) ;
#10691=ORIENTED_EDGE ( 'NONE', *, *, #3674, .F. ) ;
#10693=DIRECTION ( 'NONE',  ( -0.000000000000000000, 0.000000000000000000, -1.000000000000000000 ) ) ;
#10716=CARTESIAN_POINT ( 'NONE',  ( -18.33333333333332504, 2.000000000000000000, 7.999999999999996447 ) ) ;
#10718=ORIENTED_EDGE ( 'NONE', *, *, #3656, .T. ) ;
#10719=AXIS2_PLACEMENT_3D ( 'NONE', #848, #2830, #7922 ) ;
#10736=AXIS2_PLACEMENT_3D ( 'NONE', #6510, #7564, #5397 ) ;
#10772=ORIENTED_EDGE ( 'NONE', *, *, #3965, .F. ) ;
#10786=CARTESIAN_POINT ( 'NONE',  ( -18.33333333333332504, 30.00000000000000000, 7.999999999999996447 ) ) ;
#10791=EDGE_LOOP ( 'NONE', ( #4487, #116, #12928, #3960 ) ) ;
#10797=PLANE ( 'NONE',  #5742 ) ;
#10802=VERTEX_POINT ( 'NONE', #1794 ) ;
#10858=LINE ( 'NONE', #12894, #5415 ) ;
#10859=ORIENTED_EDGE ( 'NONE', *, *, #11997, .T. ) ;
#10863=VECTOR ( 'NONE', #357, 1000.000000000000000 ) ;
#10890=FACE_OUTER_BOUND ( 'NONE', #5176, .T. ) ;
#10894=ORIENTED_EDGE ( 'NONE', *, *, #8822, .T. ) ;
#10897=LINE ( 'NONE', #8937, #11978 ) ;
#10907=ORIENTED_EDGE ( 'NONE', *, *, #59, .F. ) ;
#10925=DIRECTION ( 'NONE',  ( 1.000000000000000000, 0.000000000000000000, -0.000000000000000000 ) ) ;
#10928=LINE ( 'NONE', #4797, #5835 ) ;
#10935=AXIS2_PLACEMENT_3D ( 'NONE', #2994, #9920, #826 ) ;
#10951=CARTESIAN_POINT ( 'NONE',  ( -64.48205080756885366, 31.76313972081441150, 1.836970198721030427E-16 ) ) ;
#10980=ORIENTED_EDGE ( 'NONE', *, *, #12332, .T. ) ;
#11027=AXIS2_PLACEMENT_3D ( 'NONE', #9622, #4905, #11104 ) ;
#11032=ORIENTED_EDGE ( 'NONE', *, *, #7530, .T. ) ;
#11051=CARTESIAN_POINT ( 'NONE',  ( -36.66666666666665009, 30.00000000000000000, 7.999999999999996447 ) ) ;
#11073=DIRECTION ( 'NONE',  ( -0.000000000000000000, 1.000000000000000000, -0.000000000000000000 ) ) ;
#11086=ORIENTED_EDGE ( 'NONE', *, *, #7435, .F. ) ;
#11087=VECTOR ( 'NONE', #8903, 1000.000000000000000 ) ;
#11100=ORIENTED_EDGE ( 'NONE', *, *, #1677, .T. ) ;
#11104=DIRECTION ( 'NONE',  ( -1.000000000000000000, 0.000000000000000000, -5.337610695313252124E-17 ) ) ;
#11106=VERTEX_POINT ( 'NONE', #9370 ) ;
#11121=EDGE_CURVE ( 'NONE', #11833, #1436, #11329, .T. ) ;
#11153=SURFACE_STYLE_USAGE ( .BOTH. , #5071 ) ;
#11161=VECTOR ( 'NONE', #2426, 1000.000000000000000 ) ;
#11167=VERTEX_POINT ( 'NONE', #1319 ) ;
#11182=VERTEX_POINT ( 'NONE', #10419 ) ;
#11189=FACE_OUTER_BOUND ( 'NONE', #12360, .T. ) ;
#11197=VECTOR ( 'NONE', #12611, 1000.000000000000000 ) ;
#11215=CARTESIAN_POINT ( 'NONE',  ( -16.33333333333332504, 46.12451549659709116, -7.999999999999996447 ) ) ;
#11220=CARTESIAN_POINT ( 'NONE',  ( -60.00000000000000000, 30.00000000000000000, -2.500000000000000000 ) ) ;
#11226=ORIENTED_EDGE ( 'NONE', *, *, #5564, .T. ) ;
#11238=DIRECTION ( 'NONE',  ( 0.000000000000000000, 0.000000000000000000, -1.000000000000000000 ) ) ;
#11239=AXIS2_PLACEMENT_3D ( 'NONE', #89, #10047, #1880 ) ;
#11240=ORIENTED_EDGE ( 'NONE', *, *, #12321, .T. ) ;
#11251=AXIS2_PLACEMENT_3D ( 'NONE', #11840, #8643, #2886 ) ;
#11263=CARTESIAN_POINT ( 'NONE',  ( -4.270088556250601699E-16, 2.000000000000000000, 8.000000000000000000 ) ) ;
#11265=ORIENTED_EDGE ( 'NONE', *, *, #5057, .F. ) ;
#11305=ORIENTED_EDGE ( 'NONE', *, *, #3674, .T. ) ;
#11313=EDGE_LOOP ( 'NONE', ( #8423, #4087, #12507, #10437 ) ) ;
#11328=AXIS2_PLACEMENT_3D ( 'NONE', #8304, #12354, #7120 ) ;
#11329=LINE ( 'NONE', #12449, #3163 ) ;
#11338=CARTESIAN_POINT ( 'NONE',  ( 5.000000000000004441, 30.00000000000000000, -10.00000000000000000 ) ) ;
#11339=CARTESIAN_POINT ( 'NONE',  ( -6.666666666666660745, 2.000000000000001332, 0.000000000000000000 ) ) ;
#11353=FACE_OUTER_BOUND ( 'NONE', #861, .T. ) ;
#11368=VECTOR ( 'NONE', #12068, 1000.000000000000000 ) ;
#11372=LINE ( 'NONE', #7454, #11161 ) ;
#11377=LINE ( 'NONE', #6278, #5198 ) ;
#11382=EDGE_CURVE ( 'NONE', #7638, #8608, #6551, .T. ) ;
#11404=CARTESIAN_POINT ( 'NONE',  ( 7.500000000000000000, 30.00000000000000000, 1.599999999999992095 ) ) ;
#11431=PLANE ( 'NONE',  #4778 ) ;
#11436=AXIS2_PLACEMENT_3D ( 'NONE', #6699, #1800, #10693 ) ;
#11453=VERTEX_POINT ( 'NONE', #11051 ) ;
#11498=ADVANCED_FACE ( 'NONE', ( #7007 ), #3812, .F. ) ;
#11509=EDGE_CURVE ( 'NONE', #7217, #3039, #4978, .T. ) ;
#11538=CARTESIAN_POINT ( 'NONE',  ( -57.99999999999999289, 2.000000000000000000, -8.000000000000003553 ) ) ;
#11542=ORIENTED_EDGE ( 'NONE', *, *, #7323, .T. ) ;
#11544=LINE ( 'NONE', #1607, #10606 ) ;
#11552=ORIENTED_EDGE ( 'NONE', *, *, #9974, .F. ) ;
#11555=VERTEX_POINT ( 'NONE', #2898 ) ;
#11568=LINE ( 'NONE', #1560, #4686 ) ;
#11582=VECTOR ( 'NONE', #4612, 1000.000000000000114 ) ;
#11586=CARTESIAN_POINT ( 'NONE',  ( -6.666666666666660745, 0.000000000000000000, 0.000000000000000000 ) ) ;
#11597=LINE ( 'NONE', #7607, #8820 ) ;
#11601=ADVANCED_FACE ( 'NONE', ( #11189 ), #6407, .T. ) ;
#11603=AXIS2_PLACEMENT_3D ( 'NONE', #9084, #3281, #7258 ) ;
#11614=CARTESIAN_POINT ( 'NONE',  ( -60.00000000000000000, 30.00000000000000000, 2.500000000000000000 ) ) ;
#11639=DIRECTION ( 'NONE',  ( 0.4999999999999985012, -0.8660254037844394848, -0.000000000000000000 ) ) ;
#11659=CARTESIAN_POINT ( 'NONE',  ( -48.33333333333332860, 0.000000000000000000, -1.599999999999998979 ) ) ;
#11666=DIRECTION ( 'NONE',  ( 0.5000000000000005551, -0.8660254037844383745, 0.000000000000000000 ) ) ;
#11667=DIRECTION ( 'NONE',  ( -0.000000000000000000, -1.000000000000000000, -0.000000000000000000 ) ) ;
#11681=AXIS2_PLACEMENT_3D ( 'NONE', #6881, #2775, #1722 ) ;
#11707=VERTEX_POINT ( 'NONE', #5300 ) ;
#11718=PLANE ( 'NONE',  #10719 ) ;
#11719=ORIENTED_EDGE ( 'NONE', *, *, #994, .T. ) ;
#11750=VERTEX_POINT ( 'NONE', #7528 ) ;
#11765=ORIENTED_EDGE ( 'NONE', *, *, #1891, .F. ) ;
#11791=MANIFOLD_SOLID_BREP ( 'M3 Clearance Hole2', #6755 ) ;
#11794=FACE_OUTER_BOUND ( 'NONE', #7244, .T. ) ;
#11817=LINE ( 'NONE', #9848, #5225 ) ;
#11818=DIRECTION ( 'NONE',  ( 0.000000000000000000, 0.000000000000000000, 1.000000000000000000 ) ) ;
#11828=PLANE ( 'NONE',  #9408 ) ;
#11833=VERTEX_POINT ( 'NONE', #7975 ) ;
#11840=CARTESIAN_POINT ( 'NONE',  ( 7.500000000000000000, 27.00000000000000000, 0.000000000000000000 ) ) ;
#11843=DIRECTION ( 'NONE',  ( -1.000000000000000000, 0.000000000000000000, 0.000000000000000000 ) ) ;
#11866=ORIENTED_EDGE ( 'NONE', *, *, #59, .T. ) ;
#11869=LINE ( 'NONE', #1000, #4759 ) ;
#11882=EDGE_LOOP ( 'NONE', ( #2948, #959, #2526, #4766 ) ) ;
#11897=ORIENTED_EDGE ( 'NONE', *, *, #12124, .T. ) ;
#11898=EDGE_CURVE ( 'NONE', #11106, #585, #6438, .T. ) ;
#11918=FACE_OUTER_BOUND ( 'NONE', #10791, .T. ) ;
#11973=MECHANICAL_DESIGN_GEOMETRIC_PRESENTATION_REPRESENTATION('',(#1945),#12609);
#11978=VECTOR ( 'NONE', #3917, 1000.000000000000000 ) ;
#11997=EDGE_CURVE ( 'NONE', #10802, #2240, #544, .T. ) ;
#12010=ORIENTED_EDGE ( 'NONE', *, *, #2964, .T. ) ;
#12042=DIRECTION ( 'NONE',  ( -0.000000000000000000, 1.000000000000000000, -0.000000000000000000 ) ) ;
#12068=DIRECTION ( 'NONE',  ( 0.000000000000000000, 0.000000000000000000, 1.000000000000000000 ) ) ;
#12071=EDGE_CURVE ( 'NONE', #946, #2543, #11597, .T. ) ;
#12079=DIRECTION ( 'NONE',  ( 1.000000000000000000, 0.000000000000000000, -0.000000000000000000 ) ) ;
#12086=ORIENTED_EDGE ( 'NONE', *, *, #5564, .F. ) ;
#12102=EDGE_CURVE ( 'NONE', #10802, #4183, #5644, .T. ) ;
#12118=DIRECTION ( 'NONE',  ( 1.000000000000000000, 0.000000000000000000, 5.337610695313252124E-17 ) ) ;
#12121=VECTOR ( 'NONE', #1085, 1000.000000000000000 ) ;
#12124=EDGE_CURVE ( 'NONE', #11182, #9021, #9864, .T. ) ;
#12127=ADVANCED_FACE ( 'NONE', ( #7672 ), #6619, .F. ) ;
#12128=VERTEX_POINT ( 'NONE', #11659 ) ;
#12136=LINE ( 'NONE', #8084, #7844 ) ;
#12143=ORIENTED_EDGE ( 'NONE', *, *, #4483, .F. ) ;
#12150=CARTESIAN_POINT ( 'NONE',  ( 5.000000000000004441, 30.00000000000000000, -2.500000000000000444 ) ) ;
#12160=FACE_OUTER_BOUND ( 'NONE', #3359, .T. ) ;
#12164=ORIENTED_EDGE ( 'NONE', *, *, #3205, .F. ) ;
#12166=DIRECTION ( 'NONE',  ( -0.000000000000000000, -1.000000000000000000, -0.000000000000000000 ) ) ;
#12172=EDGE_LOOP ( 'NONE', ( #2597, #5433, #944, #11086 ) ) ;
#12184=ORIENTED_EDGE ( 'NONE', *, *, #12198, .T. ) ;
#12197=CIRCLE ( 'NONE', #10935, 1.499999999999999778 ) ;
#12198=EDGE_CURVE ( 'NONE', #9021, #919, #9883, .T. ) ;
#12212=LINE ( 'NONE', #8220, #6982 ) ;
#12215=ORIENTED_EDGE ( 'NONE', *, *, #2897, .F. ) ;
#12224=ORIENTED_EDGE ( 'NONE', *, *, #11898, .F. ) ;
#12225=FACE_OUTER_BOUND ( 'NONE', #8896, .T. ) ;
#12229=EDGE_CURVE ( 'NONE', #4495, #8808, #3093, .T. ) ;
#12269=ADVANCED_FACE ( 'NONE', ( #915 ), #2960, .F. ) ;
#12279=CARTESIAN_POINT ( 'NONE',  ( 3.000000000000004441, 27.00000000000000000, 2.500000000000000000 ) ) ;
#12288=ADVANCED_FACE ( 'NONE', ( #3022, #7009, #1440, #1247, #381 ), #8319, .F. ) ;
#12292=VECTOR ( 'NONE', #6846, 1000.000000000000000 ) ;
#12304=CARTESIAN_POINT ( 'NONE',  ( -60.00000000000000000, 30.00000000000000000, 7.999999999999996447 ) ) ;
#12310=ORIENTED_EDGE ( 'NONE', *, *, #9909, .T. ) ;
#12321=EDGE_CURVE ( 'NONE', #10802, #7918, #2436, .T. ) ;
#12332=EDGE_CURVE ( 'NONE', #7638, #4183, #8386, .T. ) ;
#12335=ORIENTED_EDGE ( 'NONE', *, *, #10397, .F. ) ;
#12336=VECTOR ( 'NONE', #3971, 1000.000000000000227 ) ;
#12345=ORIENTED_EDGE ( 'NONE', *, *, #10397, .T. ) ;
#12348=CARTESIAN_POINT ( 'NONE',  ( -67.46410161513773573, 36.92820323027551410, -2.500000000000000000 ) ) ;
#12354=DIRECTION ( 'NONE',  ( 0.000000000000000000, -1.000000000000000000, -0.000000000000000000 ) ) ;
#12360=EDGE_LOOP ( 'NONE', ( #1312, #378, #4948, #7061 ) ) ;
#12371=AXIS2_PLACEMENT_3D ( 'NONE', #6554, #788, #5771 ) ;
#12387=ADVANCED_FACE ( 'NONE', ( #6343, #5427 ), #4328, .F. ) ;
#12394=ORIENTED_EDGE ( 'NONE', *, *, #4550, .T. ) ;
#12449=CARTESIAN_POINT ( 'NONE',  ( -48.33333333333332860, 2.000000000000000000, 1.599999999999992095 ) ) ;
#12478=CARTESIAN_POINT ( 'NONE',  ( 3.000000000000004441, 30.00000000000000000, 8.000000000000000000 ) ) ;
#12482=ORIENTED_EDGE ( 'NONE', *, *, #895, .F. ) ;
#12483=CIRCLE ( 'NONE', #3914, 1.599999999999986766 ) ;
#12503=AXIS2_PLACEMENT_3D ( 'NONE', #8692, #635, #12683 ) ;
#12507=ORIENTED_EDGE ( 'NONE', *, *, #11121, .T. ) ;
#12508=DIRECTION ( 'NONE',  ( 0.000000000000000000, 0.000000000000000000, 1.000000000000000000 ) ) ;
#12556=DIRECTION ( 'NONE',  ( -0.000000000000000000, -0.000000000000000000, -1.000000000000000000 ) ) ;
#12585=DIRECTION ( 'NONE',  ( 0.000000000000000000, 0.000000000000000000, 1.000000000000000000 ) ) ;
#12591=DIRECTION ( 'NONE',  ( 5.337610695313252124E-17, 0.000000000000000000, -1.000000000000000000 ) ) ;
#12598=CARTESIAN_POINT ( 'NONE',  ( -60.00000000000000000, 0.000000000000000000, 9.999999999999996447 ) ) ;
#12599=VERTEX_POINT ( 'NONE', #5026 ) ;
#12609=( GEOMETRIC_REPRESENTATION_CONTEXT ( 3 ) GLOBAL_UNCERTAINTY_ASSIGNED_CONTEXT ( ( #9490 ) ) GLOBAL_UNIT_ASSIGNED_CONTEXT ( ( #9260, #2276, #4169 ) ) REPRESENTATION_CONTEXT ( 'NONE', 'WORKASPACE' ) );
#12610=CARTESIAN_POINT ( 'NONE',  ( -38.66666666666665719, 46.12451549659709116, -7.999999999999996447 ) ) ;
#12611=DIRECTION ( 'NONE',  ( 0.000000000000000000, 0.000000000000000000, -1.000000000000000000 ) ) ;
#12644=ORIENTED_EDGE ( 'NONE', *, *, #6492, .F. ) ;
#12651=DIRECTION ( 'NONE',  ( -0.000000000000000000, 1.000000000000000000, -0.000000000000000000 ) ) ;
#12671=ADVANCED_FACE ( 'NONE', ( #12160 ), #6327, .T. ) ;
#12683=DIRECTION ( 'NONE',  ( 0.000000000000000000, 0.000000000000000000, 1.000000000000000000 ) ) ;
#12694=ORIENTED_EDGE ( 'NONE', *, *, #4843, .T. ) ;
#12701=CARTESIAN_POINT ( 'NONE',  ( -57.99999999999999289, 30.00000000000000000, 9.999999999999996447 ) ) ;
#12703=DIRECTION ( 'NONE',  ( -0.000000000000000000, -0.000000000000000000, -1.000000000000000000 ) ) ;
#12710=LINE ( 'NONE', #3813, #2878 ) ;
#12713=ADVANCED_FACE ( 'NONE', ( #6128, #12225 ), #1228, .T. ) ;
#12731=VECTOR ( 'NONE', #637, 1000.000000000000000 ) ;
#12743=DIRECTION ( 'NONE',  ( 0.000000000000000000, 0.000000000000000000, -1.000000000000000000 ) ) ;
#12745=CARTESIAN_POINT ( 'NONE',  ( -16.33333333333332504, 46.12451549659709116, 7.999999999999996447 ) ) ;
#12754=DIRECTION ( 'NONE',  ( -0.000000000000000000, -1.000000000000000000, -0.000000000000000000 ) ) ;
#12756=ORIENTED_EDGE ( 'NONE', *, *, #11382, .F. ) ;
#12759=CARTESIAN_POINT ( 'NONE',  ( -62.98205080756885366, 29.16506350946109194, 0.000000000000000000 ) ) ;
#12772=LINE ( 'NONE', #12832, #6618 ) ;
#12779=FACE_BOUND ( 'NONE', #8200, .T. ) ;
#12800=LINE ( 'NONE', #3843, #9340 ) ;
#12832=CARTESIAN_POINT ( 'NONE',  ( -60.00000000000000000, 30.00000000000000000, -10.00000000000000355 ) ) ;
#12848=EDGE_CURVE ( 'NONE', #11167, #3079, #8500, .T. ) ;
#12861=EDGE_CURVE ( 'NONE', #6204, #10216, #3529, .T. ) ;
#12872=PRODUCT_DEFINITION_CONTEXT ( 'detailed design', #2267, 'design' ) ;
#12890=ORIENTED_EDGE ( 'NONE', *, *, #4794, .F. ) ;
#12894=CARTESIAN_POINT ( 'NONE',  ( -63.99999999999998579, 36.92820323027551410, 2.500000000000000000 ) ) ;
#12895=ORIENTED_EDGE ( 'NONE', *, *, #4844, .F. ) ;
#12905=FACE_BOUND ( 'NONE', #9231, .T. ) ;
#12909=AXIS2_PLACEMENT_3D ( 'NONE', #7270, #6085, #6020 ) ;
#12924=CARTESIAN_POINT ( 'NONE',  ( -60.00000000000000000, 23.99999999999998934, -2.500000000000000000 ) ) ;
#12927=CARTESIAN_POINT ( 'NONE',  ( -6.666666666666660745, 2.000000000000001332, 0.000000000000000000 ) ) ;
#12928=ORIENTED_EDGE ( 'NONE', *, *, #1486, .F. ) ;
#12944=DIRECTION ( 'NONE',  ( 0.000000000000000000, 0.000000000000000000, 1.000000000000000000 ) ) ;
#12948=ORIENTED_EDGE ( 'NONE', *, *, #9639, .T. ) ;
#12989=COLOUR_RGB('Sky Blue',0.24,0.69,0.87);
#12990=FILL_AREA_STYLE_COLOUR('',#12989);
#12991=FILL_AREA_STYLE('',(#12990));
#12992=SURFACE_STYLE_FILL_AREA(#12991);
#12993=SURFACE_SIDE_STYLE('',(#12992));
#12994=SURFACE_STYLE_USAGE(.BOTH.,#12993);
#12995=PRESENTATION_STYLE_ASSIGNMENT((#12994));
ENDSEC;
END-ISO-10303-21;
